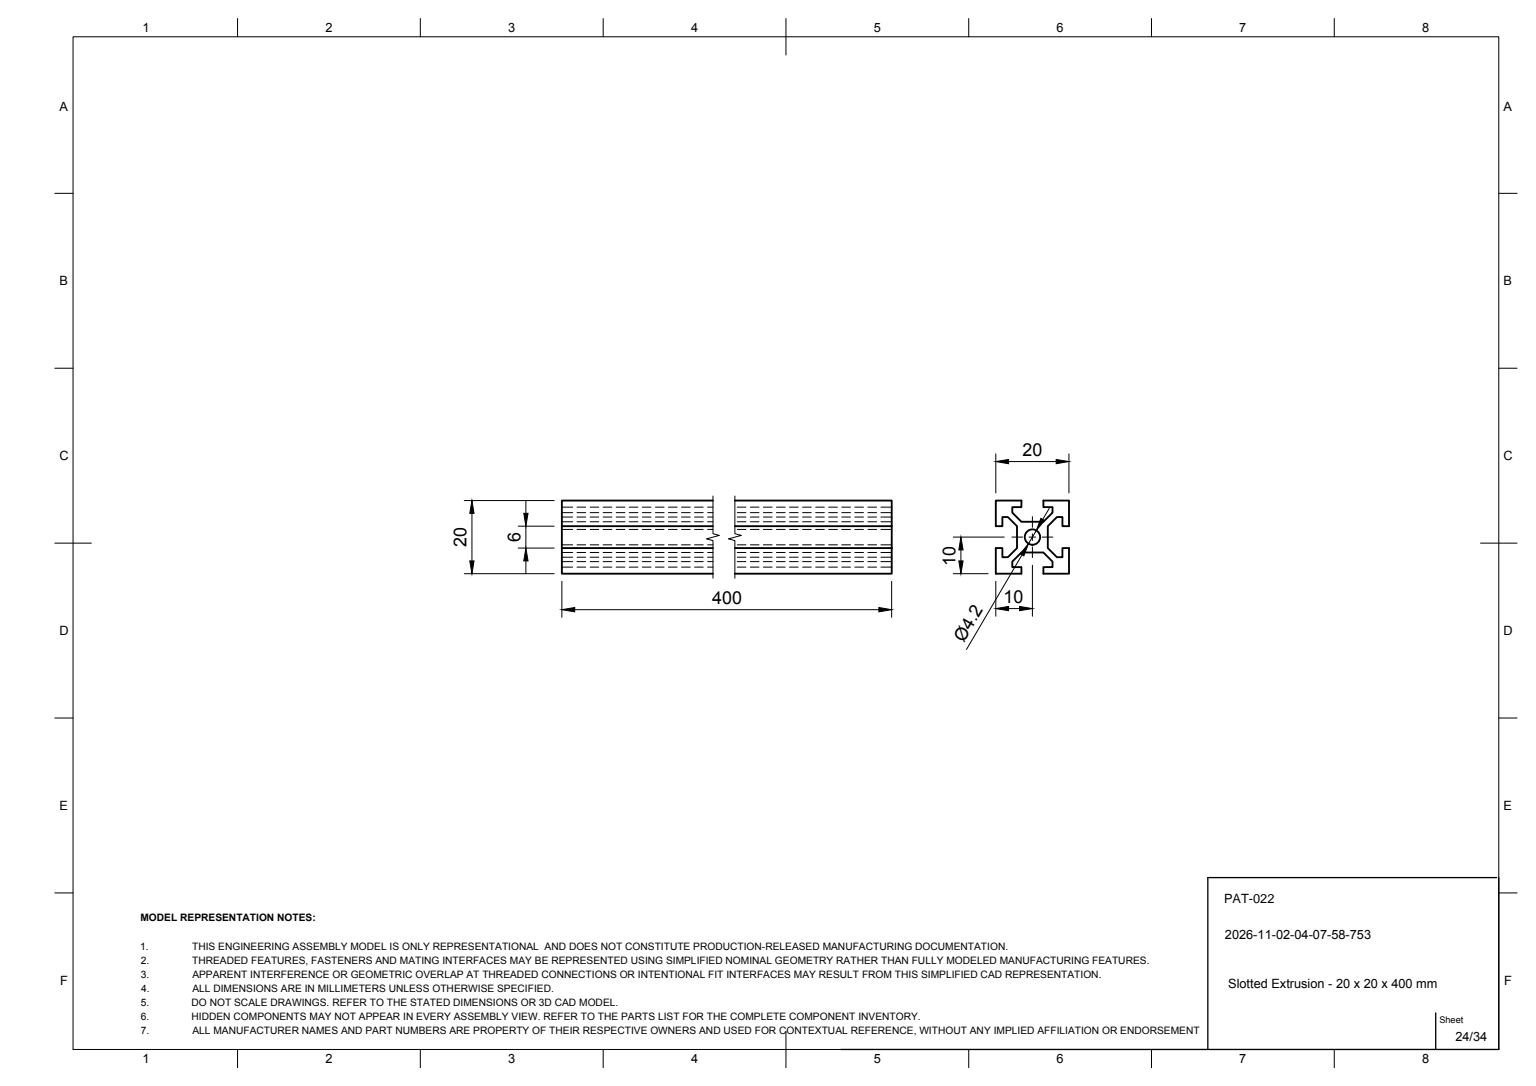
ISO-10303-21;
HEADER;
/* Generated by software containing ST-Developer
 * from STEP Tools, Inc. (www.steptools.com) 
 */

FILE_DESCRIPTION(
/* description */ ('Chute with adjustable gate'),
/* implementation_level */ '2;1');

FILE_NAME(
/* name */ 'Slotted Extrusion - 20 x 20 x 400 mm.step',
/* time_stamp */ '2026-10-27T10:52:28-07:00',
/* author */ (''),
/* organization */ (''),
/* preprocessor_version */ 'ST-DEVELOPER v20.2',
/* originating_system */ 'Autodesk Translation Framework v15.17.0.0',
/* authorisation */ '');

FILE_SCHEMA (('AUTOMOTIVE_DESIGN { 1 0 10303 214 3 1 1 }'));
ENDSEC;

DATA;
#10=MECHANICAL_DESIGN_GEOMETRIC_PRESENTATION_REPRESENTATION('',(#433),#13094);
#369=SHAPE_REPRESENTATION_RELATIONSHIP('SRR','None',#13270,#401);
#401=ADVANCED_BREP_SHAPE_REPRESENTATION('',(#465),#13079);
#433=STYLED_ITEM('',(#13481),#465);
#465=MANIFOLD_SOLID_BREP('Body1',#7616);
#550=FACE_BOUND('',#1635,.T.);
#551=FACE_BOUND('',#1637,.T.);
#734=PLANE('',#8272);
#735=PLANE('',#8273);
#736=PLANE('',#8274);
#737=PLANE('',#8275);
#738=PLANE('',#8276);
#739=PLANE('',#8277);
#740=PLANE('',#8278);
#741=PLANE('',#8279);
#742=PLANE('',#8280);
#743=PLANE('',#8281);
#744=PLANE('',#8282);
#745=PLANE('',#8283);
#746=PLANE('',#8284);
#747=PLANE('',#8285);
#748=PLANE('',#8286);
#749=PLANE('',#8287);
#750=PLANE('',#8288);
#751=PLANE('',#8289);
#752=PLANE('',#8290);
#753=PLANE('',#8291);
#754=PLANE('',#8292);
#755=PLANE('',#8293);
#756=PLANE('',#8294);
#757=PLANE('',#8295);
#758=PLANE('',#8296);
#759=PLANE('',#8297);
#760=PLANE('',#8298);
#761=PLANE('',#8299);
#762=PLANE('',#8300);
#763=PLANE('',#8301);
#764=PLANE('',#8302);
#765=PLANE('',#8303);
#766=PLANE('',#8304);
#767=PLANE('',#8305);
#768=PLANE('',#8306);
#769=PLANE('',#8307);
#770=PLANE('',#8311);
#771=PLANE('',#8312);
#772=PLANE('',#8313);
#773=PLANE('',#8314);
#774=PLANE('',#8315);
#775=PLANE('',#8316);
#776=PLANE('',#8317);
#777=PLANE('',#8318);
#778=PLANE('',#8319);
#779=PLANE('',#8320);
#1098=FACE_OUTER_BOUND('',#1589,.T.);
#1099=FACE_OUTER_BOUND('',#1590,.T.);
#1100=FACE_OUTER_BOUND('',#1591,.T.);
#1101=FACE_OUTER_BOUND('',#1592,.T.);
#1102=FACE_OUTER_BOUND('',#1593,.T.);
#1103=FACE_OUTER_BOUND('',#1594,.T.);
#1104=FACE_OUTER_BOUND('',#1595,.T.);
#1105=FACE_OUTER_BOUND('',#1596,.T.);
#1106=FACE_OUTER_BOUND('',#1597,.T.);
#1107=FACE_OUTER_BOUND('',#1598,.T.);
#1108=FACE_OUTER_BOUND('',#1599,.T.);
#1109=FACE_OUTER_BOUND('',#1600,.T.);
#1110=FACE_OUTER_BOUND('',#1601,.T.);
#1111=FACE_OUTER_BOUND('',#1602,.T.);
#1112=FACE_OUTER_BOUND('',#1603,.T.);
#1113=FACE_OUTER_BOUND('',#1604,.T.);
#1114=FACE_OUTER_BOUND('',#1605,.T.);
#1115=FACE_OUTER_BOUND('',#1606,.T.);
#1116=FACE_OUTER_BOUND('',#1607,.T.);
#1117=FACE_OUTER_BOUND('',#1608,.T.);
#1118=FACE_OUTER_BOUND('',#1609,.T.);
#1119=FACE_OUTER_BOUND('',#1610,.T.);
#1120=FACE_OUTER_BOUND('',#1611,.T.);
#1121=FACE_OUTER_BOUND('',#1612,.T.);
#1122=FACE_OUTER_BOUND('',#1613,.T.);
#1123=FACE_OUTER_BOUND('',#1614,.T.);
#1124=FACE_OUTER_BOUND('',#1615,.T.);
#1125=FACE_OUTER_BOUND('',#1616,.T.);
#1126=FACE_OUTER_BOUND('',#1617,.T.);
#1127=FACE_OUTER_BOUND('',#1618,.T.);
#1128=FACE_OUTER_BOUND('',#1619,.T.);
#1129=FACE_OUTER_BOUND('',#1620,.T.);
#1130=FACE_OUTER_BOUND('',#1621,.T.);
#1131=FACE_OUTER_BOUND('',#1622,.T.);
#1132=FACE_OUTER_BOUND('',#1623,.T.);
#1133=FACE_OUTER_BOUND('',#1624,.T.);
#1134=FACE_OUTER_BOUND('',#1625,.T.);
#1135=FACE_OUTER_BOUND('',#1626,.T.);
#1136=FACE_OUTER_BOUND('',#1627,.T.);
#1137=FACE_OUTER_BOUND('',#1628,.T.);
#1138=FACE_OUTER_BOUND('',#1629,.T.);
#1139=FACE_OUTER_BOUND('',#1630,.T.);
#1140=FACE_OUTER_BOUND('',#1631,.T.);
#1141=FACE_OUTER_BOUND('',#1632,.T.);
#1142=FACE_OUTER_BOUND('',#1633,.T.);
#1143=FACE_OUTER_BOUND('',#1634,.T.);
#1144=FACE_OUTER_BOUND('',#1636,.T.);
#1589=EDGE_LOOP('',(#6002,#6003,#6004,#6005));
#1590=EDGE_LOOP('',(#6006,#6007,#6008,#6009));
#1591=EDGE_LOOP('',(#6010,#6011,#6012,#6013));
#1592=EDGE_LOOP('',(#6014,#6015,#6016,#6017));
#1593=EDGE_LOOP('',(#6018,#6019,#6020,#6021));
#1594=EDGE_LOOP('',(#6022,#6023,#6024,#6025));
#1595=EDGE_LOOP('',(#6026,#6027,#6028,#6029));
#1596=EDGE_LOOP('',(#6030,#6031,#6032,#6033));
#1597=EDGE_LOOP('',(#6034,#6035,#6036,#6037));
#1598=EDGE_LOOP('',(#6038,#6039,#6040,#6041));
#1599=EDGE_LOOP('',(#6042,#6043,#6044,#6045));
#1600=EDGE_LOOP('',(#6046,#6047,#6048,#6049));
#1601=EDGE_LOOP('',(#6050,#6051,#6052,#6053));
#1602=EDGE_LOOP('',(#6054,#6055,#6056,#6057));
#1603=EDGE_LOOP('',(#6058,#6059,#6060,#6061));
#1604=EDGE_LOOP('',(#6062,#6063,#6064,#6065));
#1605=EDGE_LOOP('',(#6066,#6067,#6068,#6069));
#1606=EDGE_LOOP('',(#6070,#6071,#6072,#6073));
#1607=EDGE_LOOP('',(#6074,#6075,#6076,#6077));
#1608=EDGE_LOOP('',(#6078,#6079,#6080,#6081));
#1609=EDGE_LOOP('',(#6082,#6083,#6084,#6085));
#1610=EDGE_LOOP('',(#6086,#6087,#6088,#6089));
#1611=EDGE_LOOP('',(#6090,#6091,#6092,#6093));
#1612=EDGE_LOOP('',(#6094,#6095,#6096,#6097));
#1613=EDGE_LOOP('',(#6098,#6099,#6100,#6101));
#1614=EDGE_LOOP('',(#6102,#6103,#6104,#6105));
#1615=EDGE_LOOP('',(#6106,#6107,#6108,#6109));
#1616=EDGE_LOOP('',(#6110,#6111,#6112,#6113));
#1617=EDGE_LOOP('',(#6114,#6115,#6116,#6117));
#1618=EDGE_LOOP('',(#6118,#6119,#6120,#6121));
#1619=EDGE_LOOP('',(#6122,#6123,#6124,#6125));
#1620=EDGE_LOOP('',(#6126,#6127,#6128,#6129));
#1621=EDGE_LOOP('',(#6130,#6131,#6132,#6133));
#1622=EDGE_LOOP('',(#6134,#6135,#6136,#6137));
#1623=EDGE_LOOP('',(#6138,#6139,#6140,#6141));
#1624=EDGE_LOOP('',(#6142,#6143,#6144,#6145));
#1625=EDGE_LOOP('',(#6146,#6147,#6148,#6149));
#1626=EDGE_LOOP('',(#6150,#6151,#6152,#6153));
#1627=EDGE_LOOP('',(#6154,#6155,#6156,#6157));
#1628=EDGE_LOOP('',(#6158,#6159,#6160,#6161));
#1629=EDGE_LOOP('',(#6162,#6163,#6164,#6165));
#1630=EDGE_LOOP('',(#6166,#6167,#6168,#6169));
#1631=EDGE_LOOP('',(#6170,#6171,#6172,#6173));
#1632=EDGE_LOOP('',(#6174,#6175,#6176,#6177));
#1633=EDGE_LOOP('',(#6178,#6179,#6180,#6181));
#1634=EDGE_LOOP('',(#6182,#6183,#6184,#6185,#6186,#6187,#6188,#6189,#6190,
#6191,#6192,#6193,#6194,#6195,#6196,#6197,#6198,#6199,#6200,#6201,#6202,
#6203,#6204,#6205,#6206,#6207,#6208,#6209,#6210,#6211,#6212,#6213,#6214,
#6215,#6216,#6217,#6218,#6219,#6220,#6221,#6222,#6223,#6224,#6225));
#1635=EDGE_LOOP('',(#6226));
#1636=EDGE_LOOP('',(#6227,#6228,#6229,#6230,#6231,#6232,#6233,#6234,#6235,
#6236,#6237,#6238,#6239,#6240,#6241,#6242,#6243,#6244,#6245,#6246,#6247,
#6248,#6249,#6250,#6251,#6252,#6253,#6254,#6255,#6256,#6257,#6258,#6259,
#6260,#6261,#6262,#6263,#6264,#6265,#6266,#6267,#6268,#6269,#6270));
#1637=EDGE_LOOP('',(#6271));
#2188=LINE('',#11788,#2965);
#2189=LINE('',#11790,#2966);
#2190=LINE('',#11792,#2967);
#2191=LINE('',#11793,#2968);
#2192=LINE('',#11796,#2969);
#2193=LINE('',#11798,#2970);
#2194=LINE('',#11799,#2971);
#2195=LINE('',#11802,#2972);
#2196=LINE('',#11804,#2973);
#2197=LINE('',#11805,#2974);
#2198=LINE('',#11808,#2975);
#2199=LINE('',#11810,#2976);
#2200=LINE('',#11811,#2977);
#2201=LINE('',#11814,#2978);
#2202=LINE('',#11816,#2979);
#2203=LINE('',#11817,#2980);
#2204=LINE('',#11820,#2981);
#2205=LINE('',#11822,#2982);
#2206=LINE('',#11823,#2983);
#2207=LINE('',#11826,#2984);
#2208=LINE('',#11828,#2985);
#2209=LINE('',#11829,#2986);
#2210=LINE('',#11832,#2987);
#2211=LINE('',#11834,#2988);
#2212=LINE('',#11835,#2989);
#2213=LINE('',#11838,#2990);
#2214=LINE('',#11840,#2991);
#2215=LINE('',#11841,#2992);
#2216=LINE('',#11845,#2993);
#2217=LINE('',#11847,#2994);
#2218=LINE('',#11849,#2995);
#2219=LINE('',#11850,#2996);
#2220=LINE('',#11853,#2997);
#2221=LINE('',#11855,#2998);
#2222=LINE('',#11856,#2999);
#2223=LINE('',#11859,#3000);
#2224=LINE('',#11861,#3001);
#2225=LINE('',#11862,#3002);
#2226=LINE('',#11865,#3003);
#2227=LINE('',#11867,#3004);
#2228=LINE('',#11868,#3005);
#2229=LINE('',#11871,#3006);
#2230=LINE('',#11873,#3007);
#2231=LINE('',#11874,#3008);
#2232=LINE('',#11877,#3009);
#2233=LINE('',#11879,#3010);
#2234=LINE('',#11880,#3011);
#2235=LINE('',#11883,#3012);
#2236=LINE('',#11885,#3013);
#2237=LINE('',#11886,#3014);
#2238=LINE('',#11889,#3015);
#2239=LINE('',#11891,#3016);
#2240=LINE('',#11892,#3017);
#2241=LINE('',#11895,#3018);
#2242=LINE('',#11897,#3019);
#2243=LINE('',#11898,#3020);
#2244=LINE('',#11902,#3021);
#2245=LINE('',#11904,#3022);
#2246=LINE('',#11906,#3023);
#2247=LINE('',#11907,#3024);
#2248=LINE('',#11910,#3025);
#2249=LINE('',#11912,#3026);
#2250=LINE('',#11913,#3027);
#2251=LINE('',#11916,#3028);
#2252=LINE('',#11918,#3029);
#2253=LINE('',#11919,#3030);
#2254=LINE('',#11922,#3031);
#2255=LINE('',#11924,#3032);
#2256=LINE('',#11925,#3033);
#2257=LINE('',#11928,#3034);
#2258=LINE('',#11930,#3035);
#2259=LINE('',#11931,#3036);
#2260=LINE('',#11934,#3037);
#2261=LINE('',#11936,#3038);
#2262=LINE('',#11937,#3039);
#2263=LINE('',#11940,#3040);
#2264=LINE('',#11942,#3041);
#2265=LINE('',#11943,#3042);
#2266=LINE('',#11946,#3043);
#2267=LINE('',#11948,#3044);
#2268=LINE('',#11949,#3045);
#2269=LINE('',#11952,#3046);
#2270=LINE('',#11954,#3047);
#2271=LINE('',#11955,#3048);
#2272=LINE('',#11959,#3049);
#2273=LINE('',#11961,#3050);
#2274=LINE('',#11963,#3051);
#2275=LINE('',#11964,#3052);
#2276=LINE('',#11967,#3053);
#2277=LINE('',#11969,#3054);
#2278=LINE('',#11970,#3055);
#2279=LINE('',#11973,#3056);
#2280=LINE('',#11975,#3057);
#2281=LINE('',#11976,#3058);
#2282=LINE('',#11979,#3059);
#2283=LINE('',#11981,#3060);
#2284=LINE('',#11982,#3061);
#2285=LINE('',#11985,#3062);
#2286=LINE('',#11987,#3063);
#2287=LINE('',#11988,#3064);
#2288=LINE('',#11991,#3065);
#2289=LINE('',#11993,#3066);
#2290=LINE('',#11994,#3067);
#2291=LINE('',#11997,#3068);
#2292=LINE('',#11999,#3069);
#2293=LINE('',#12000,#3070);
#2294=LINE('',#12003,#3071);
#2295=LINE('',#12005,#3072);
#2296=LINE('',#12006,#3073);
#2297=LINE('',#12009,#3074);
#2298=LINE('',#12011,#3075);
#2299=LINE('',#12012,#3076);
#2300=LINE('',#12017,#3077);
#2301=LINE('',#12021,#3078);
#2302=LINE('',#12023,#3079);
#2303=LINE('',#12024,#3080);
#2304=LINE('',#12027,#3081);
#2305=LINE('',#12029,#3082);
#2306=LINE('',#12030,#3083);
#2307=LINE('',#12032,#3084);
#2308=LINE('',#12033,#3085);
#2309=LINE('',#12036,#3086);
#2310=LINE('',#12038,#3087);
#2311=LINE('',#12039,#3088);
#2312=LINE('',#12041,#3089);
#2313=LINE('',#12042,#3090);
#2314=LINE('',#12045,#3091);
#2315=LINE('',#12047,#3092);
#2316=LINE('',#12048,#3093);
#2317=LINE('',#12050,#3094);
#2318=LINE('',#12051,#3095);
#2319=LINE('',#12053,#3096);
#2320=LINE('',#12054,#3097);
#2965=VECTOR('',#9600,1.);
#2966=VECTOR('',#9601,1.);
#2967=VECTOR('',#9602,1.);
#2968=VECTOR('',#9603,1.);
#2969=VECTOR('',#9606,1.);
#2970=VECTOR('',#9607,1.);
#2971=VECTOR('',#9608,1.);
#2972=VECTOR('',#9611,1.);
#2973=VECTOR('',#9612,1.);
#2974=VECTOR('',#9613,1.);
#2975=VECTOR('',#9616,1.);
#2976=VECTOR('',#9617,1.);
#2977=VECTOR('',#9618,1.);
#2978=VECTOR('',#9621,1.);
#2979=VECTOR('',#9622,1.);
#2980=VECTOR('',#9623,1.);
#2981=VECTOR('',#9626,1.);
#2982=VECTOR('',#9627,1.);
#2983=VECTOR('',#9628,1.);
#2984=VECTOR('',#9631,1.);
#2985=VECTOR('',#9632,1.);
#2986=VECTOR('',#9633,1.);
#2987=VECTOR('',#9636,1.);
#2988=VECTOR('',#9637,1.);
#2989=VECTOR('',#9638,1.);
#2990=VECTOR('',#9641,1.);
#2991=VECTOR('',#9642,1.);
#2992=VECTOR('',#9643,1.);
#2993=VECTOR('',#9646,1.);
#2994=VECTOR('',#9647,1.);
#2995=VECTOR('',#9648,1.);
#2996=VECTOR('',#9649,1.);
#2997=VECTOR('',#9652,1.);
#2998=VECTOR('',#9653,1.);
#2999=VECTOR('',#9654,1.);
#3000=VECTOR('',#9657,1.);
#3001=VECTOR('',#9658,1.);
#3002=VECTOR('',#9659,1.);
#3003=VECTOR('',#9662,1.);
#3004=VECTOR('',#9663,1.);
#3005=VECTOR('',#9664,1.);
#3006=VECTOR('',#9667,1.);
#3007=VECTOR('',#9668,1.);
#3008=VECTOR('',#9669,1.);
#3009=VECTOR('',#9672,1.);
#3010=VECTOR('',#9673,1.);
#3011=VECTOR('',#9674,1.);
#3012=VECTOR('',#9677,1.);
#3013=VECTOR('',#9678,1.);
#3014=VECTOR('',#9679,1.);
#3015=VECTOR('',#9682,1.);
#3016=VECTOR('',#9683,1.);
#3017=VECTOR('',#9684,1.);
#3018=VECTOR('',#9687,1.);
#3019=VECTOR('',#9688,1.);
#3020=VECTOR('',#9689,1.);
#3021=VECTOR('',#9692,1.);
#3022=VECTOR('',#9693,1.);
#3023=VECTOR('',#9694,1.);
#3024=VECTOR('',#9695,1.);
#3025=VECTOR('',#9698,1.);
#3026=VECTOR('',#9699,1.);
#3027=VECTOR('',#9700,1.);
#3028=VECTOR('',#9703,1.);
#3029=VECTOR('',#9704,1.);
#3030=VECTOR('',#9705,1.);
#3031=VECTOR('',#9708,1.);
#3032=VECTOR('',#9709,1.);
#3033=VECTOR('',#9710,1.);
#3034=VECTOR('',#9713,1.);
#3035=VECTOR('',#9714,1.);
#3036=VECTOR('',#9715,1.);
#3037=VECTOR('',#9718,1.);
#3038=VECTOR('',#9719,1.);
#3039=VECTOR('',#9720,1.);
#3040=VECTOR('',#9723,1.);
#3041=VECTOR('',#9724,1.);
#3042=VECTOR('',#9725,1.);
#3043=VECTOR('',#9728,1.);
#3044=VECTOR('',#9729,1.);
#3045=VECTOR('',#9730,1.);
#3046=VECTOR('',#9733,1.);
#3047=VECTOR('',#9734,1.);
#3048=VECTOR('',#9735,1.);
#3049=VECTOR('',#9738,1.);
#3050=VECTOR('',#9739,1.);
#3051=VECTOR('',#9740,1.);
#3052=VECTOR('',#9741,1.);
#3053=VECTOR('',#9744,1.);
#3054=VECTOR('',#9745,1.);
#3055=VECTOR('',#9746,1.);
#3056=VECTOR('',#9749,1.);
#3057=VECTOR('',#9750,1.);
#3058=VECTOR('',#9751,1.);
#3059=VECTOR('',#9754,1.);
#3060=VECTOR('',#9755,1.);
#3061=VECTOR('',#9756,1.);
#3062=VECTOR('',#9759,1.);
#3063=VECTOR('',#9760,1.);
#3064=VECTOR('',#9761,1.);
#3065=VECTOR('',#9764,1.);
#3066=VECTOR('',#9765,1.);
#3067=VECTOR('',#9766,1.);
#3068=VECTOR('',#9769,1.);
#3069=VECTOR('',#9770,1.);
#3070=VECTOR('',#9771,1.);
#3071=VECTOR('',#9774,1.);
#3072=VECTOR('',#9775,1.);
#3073=VECTOR('',#9776,1.);
#3074=VECTOR('',#9779,1.);
#3075=VECTOR('',#9780,1.);
#3076=VECTOR('',#9781,1.);
#3077=VECTOR('',#9786,0.21);
#3078=VECTOR('',#9791,1.);
#3079=VECTOR('',#9792,1.);
#3080=VECTOR('',#9793,1.);
#3081=VECTOR('',#9796,1.);
#3082=VECTOR('',#9797,1.);
#3083=VECTOR('',#9798,1.);
#3084=VECTOR('',#9801,1.);
#3085=VECTOR('',#9802,1.);
#3086=VECTOR('',#9805,1.);
#3087=VECTOR('',#9806,1.);
#3088=VECTOR('',#9807,1.);
#3089=VECTOR('',#9810,1.);
#3090=VECTOR('',#9811,1.);
#3091=VECTOR('',#9814,1.);
#3092=VECTOR('',#9815,1.);
#3093=VECTOR('',#9816,1.);
#3094=VECTOR('',#9819,1.);
#3095=VECTOR('',#9820,1.);
#3096=VECTOR('',#9823,1.);
#3097=VECTOR('',#9824,1.);
#3494=CIRCLE('',#8309,0.21);
#3495=CIRCLE('',#8310,0.21);
#3865=VERTEX_POINT('',#11786);
#3866=VERTEX_POINT('',#11787);
#3867=VERTEX_POINT('',#11789);
#3868=VERTEX_POINT('',#11791);
#3869=VERTEX_POINT('',#11795);
#3870=VERTEX_POINT('',#11797);
#3871=VERTEX_POINT('',#11801);
#3872=VERTEX_POINT('',#11803);
#3873=VERTEX_POINT('',#11807);
#3874=VERTEX_POINT('',#11809);
#3875=VERTEX_POINT('',#11813);
#3876=VERTEX_POINT('',#11815);
#3877=VERTEX_POINT('',#11819);
#3878=VERTEX_POINT('',#11821);
#3879=VERTEX_POINT('',#11825);
#3880=VERTEX_POINT('',#11827);
#3881=VERTEX_POINT('',#11831);
#3882=VERTEX_POINT('',#11833);
#3883=VERTEX_POINT('',#11837);
#3884=VERTEX_POINT('',#11839);
#3885=VERTEX_POINT('',#11843);
#3886=VERTEX_POINT('',#11844);
#3887=VERTEX_POINT('',#11846);
#3888=VERTEX_POINT('',#11848);
#3889=VERTEX_POINT('',#11852);
#3890=VERTEX_POINT('',#11854);
#3891=VERTEX_POINT('',#11858);
#3892=VERTEX_POINT('',#11860);
#3893=VERTEX_POINT('',#11864);
#3894=VERTEX_POINT('',#11866);
#3895=VERTEX_POINT('',#11870);
#3896=VERTEX_POINT('',#11872);
#3897=VERTEX_POINT('',#11876);
#3898=VERTEX_POINT('',#11878);
#3899=VERTEX_POINT('',#11882);
#3900=VERTEX_POINT('',#11884);
#3901=VERTEX_POINT('',#11888);
#3902=VERTEX_POINT('',#11890);
#3903=VERTEX_POINT('',#11894);
#3904=VERTEX_POINT('',#11896);
#3905=VERTEX_POINT('',#11900);
#3906=VERTEX_POINT('',#11901);
#3907=VERTEX_POINT('',#11903);
#3908=VERTEX_POINT('',#11905);
#3909=VERTEX_POINT('',#11909);
#3910=VERTEX_POINT('',#11911);
#3911=VERTEX_POINT('',#11915);
#3912=VERTEX_POINT('',#11917);
#3913=VERTEX_POINT('',#11921);
#3914=VERTEX_POINT('',#11923);
#3915=VERTEX_POINT('',#11927);
#3916=VERTEX_POINT('',#11929);
#3917=VERTEX_POINT('',#11933);
#3918=VERTEX_POINT('',#11935);
#3919=VERTEX_POINT('',#11939);
#3920=VERTEX_POINT('',#11941);
#3921=VERTEX_POINT('',#11945);
#3922=VERTEX_POINT('',#11947);
#3923=VERTEX_POINT('',#11951);
#3924=VERTEX_POINT('',#11953);
#3925=VERTEX_POINT('',#11957);
#3926=VERTEX_POINT('',#11958);
#3927=VERTEX_POINT('',#11960);
#3928=VERTEX_POINT('',#11962);
#3929=VERTEX_POINT('',#11966);
#3930=VERTEX_POINT('',#11968);
#3931=VERTEX_POINT('',#11972);
#3932=VERTEX_POINT('',#11974);
#3933=VERTEX_POINT('',#11978);
#3934=VERTEX_POINT('',#11980);
#3935=VERTEX_POINT('',#11984);
#3936=VERTEX_POINT('',#11986);
#3937=VERTEX_POINT('',#11990);
#3938=VERTEX_POINT('',#11992);
#3939=VERTEX_POINT('',#11996);
#3940=VERTEX_POINT('',#11998);
#3941=VERTEX_POINT('',#12002);
#3942=VERTEX_POINT('',#12004);
#3943=VERTEX_POINT('',#12008);
#3944=VERTEX_POINT('',#12010);
#3945=VERTEX_POINT('',#12014);
#3946=VERTEX_POINT('',#12016);
#3947=VERTEX_POINT('',#12020);
#3948=VERTEX_POINT('',#12022);
#3949=VERTEX_POINT('',#12026);
#3950=VERTEX_POINT('',#12028);
#3951=VERTEX_POINT('',#12035);
#3952=VERTEX_POINT('',#12037);
#3953=VERTEX_POINT('',#12044);
#3954=VERTEX_POINT('',#12046);
#4634=EDGE_CURVE('',#3865,#3866,#2188,.T.);
#4635=EDGE_CURVE('',#3865,#3867,#2189,.T.);
#4636=EDGE_CURVE('',#3868,#3867,#2190,.T.);
#4637=EDGE_CURVE('',#3866,#3868,#2191,.T.);
#4638=EDGE_CURVE('',#3869,#3865,#2192,.T.);
#4639=EDGE_CURVE('',#3869,#3870,#2193,.T.);
#4640=EDGE_CURVE('',#3867,#3870,#2194,.T.);
#4641=EDGE_CURVE('',#3871,#3869,#2195,.T.);
#4642=EDGE_CURVE('',#3871,#3872,#2196,.T.);
#4643=EDGE_CURVE('',#3870,#3872,#2197,.T.);
#4644=EDGE_CURVE('',#3873,#3871,#2198,.T.);
#4645=EDGE_CURVE('',#3873,#3874,#2199,.T.);
#4646=EDGE_CURVE('',#3872,#3874,#2200,.T.);
#4647=EDGE_CURVE('',#3875,#3873,#2201,.T.);
#4648=EDGE_CURVE('',#3875,#3876,#2202,.T.);
#4649=EDGE_CURVE('',#3874,#3876,#2203,.T.);
#4650=EDGE_CURVE('',#3877,#3875,#2204,.T.);
#4651=EDGE_CURVE('',#3877,#3878,#2205,.T.);
#4652=EDGE_CURVE('',#3876,#3878,#2206,.T.);
#4653=EDGE_CURVE('',#3879,#3877,#2207,.T.);
#4654=EDGE_CURVE('',#3879,#3880,#2208,.T.);
#4655=EDGE_CURVE('',#3878,#3880,#2209,.T.);
#4656=EDGE_CURVE('',#3881,#3879,#2210,.T.);
#4657=EDGE_CURVE('',#3881,#3882,#2211,.T.);
#4658=EDGE_CURVE('',#3880,#3882,#2212,.T.);
#4659=EDGE_CURVE('',#3883,#3881,#2213,.T.);
#4660=EDGE_CURVE('',#3884,#3883,#2214,.T.);
#4661=EDGE_CURVE('',#3882,#3884,#2215,.T.);
#4662=EDGE_CURVE('',#3885,#3886,#2216,.T.);
#4663=EDGE_CURVE('',#3885,#3887,#2217,.T.);
#4664=EDGE_CURVE('',#3888,#3887,#2218,.T.);
#4665=EDGE_CURVE('',#3886,#3888,#2219,.T.);
#4666=EDGE_CURVE('',#3889,#3885,#2220,.T.);
#4667=EDGE_CURVE('',#3889,#3890,#2221,.T.);
#4668=EDGE_CURVE('',#3887,#3890,#2222,.T.);
#4669=EDGE_CURVE('',#3891,#3889,#2223,.T.);
#4670=EDGE_CURVE('',#3891,#3892,#2224,.T.);
#4671=EDGE_CURVE('',#3890,#3892,#2225,.T.);
#4672=EDGE_CURVE('',#3893,#3891,#2226,.T.);
#4673=EDGE_CURVE('',#3893,#3894,#2227,.T.);
#4674=EDGE_CURVE('',#3892,#3894,#2228,.T.);
#4675=EDGE_CURVE('',#3895,#3893,#2229,.T.);
#4676=EDGE_CURVE('',#3895,#3896,#2230,.T.);
#4677=EDGE_CURVE('',#3894,#3896,#2231,.T.);
#4678=EDGE_CURVE('',#3897,#3895,#2232,.T.);
#4679=EDGE_CURVE('',#3897,#3898,#2233,.T.);
#4680=EDGE_CURVE('',#3896,#3898,#2234,.T.);
#4681=EDGE_CURVE('',#3899,#3897,#2235,.T.);
#4682=EDGE_CURVE('',#3899,#3900,#2236,.T.);
#4683=EDGE_CURVE('',#3898,#3900,#2237,.T.);
#4684=EDGE_CURVE('',#3901,#3899,#2238,.T.);
#4685=EDGE_CURVE('',#3901,#3902,#2239,.T.);
#4686=EDGE_CURVE('',#3900,#3902,#2240,.T.);
#4687=EDGE_CURVE('',#3903,#3901,#2241,.T.);
#4688=EDGE_CURVE('',#3904,#3903,#2242,.T.);
#4689=EDGE_CURVE('',#3902,#3904,#2243,.T.);
#4690=EDGE_CURVE('',#3905,#3906,#2244,.T.);
#4691=EDGE_CURVE('',#3905,#3907,#2245,.T.);
#4692=EDGE_CURVE('',#3908,#3907,#2246,.T.);
#4693=EDGE_CURVE('',#3906,#3908,#2247,.T.);
#4694=EDGE_CURVE('',#3909,#3905,#2248,.T.);
#4695=EDGE_CURVE('',#3909,#3910,#2249,.T.);
#4696=EDGE_CURVE('',#3907,#3910,#2250,.T.);
#4697=EDGE_CURVE('',#3911,#3909,#2251,.T.);
#4698=EDGE_CURVE('',#3911,#3912,#2252,.T.);
#4699=EDGE_CURVE('',#3910,#3912,#2253,.T.);
#4700=EDGE_CURVE('',#3913,#3911,#2254,.T.);
#4701=EDGE_CURVE('',#3913,#3914,#2255,.T.);
#4702=EDGE_CURVE('',#3912,#3914,#2256,.T.);
#4703=EDGE_CURVE('',#3915,#3913,#2257,.T.);
#4704=EDGE_CURVE('',#3915,#3916,#2258,.T.);
#4705=EDGE_CURVE('',#3914,#3916,#2259,.T.);
#4706=EDGE_CURVE('',#3917,#3915,#2260,.T.);
#4707=EDGE_CURVE('',#3917,#3918,#2261,.T.);
#4708=EDGE_CURVE('',#3916,#3918,#2262,.T.);
#4709=EDGE_CURVE('',#3919,#3917,#2263,.T.);
#4710=EDGE_CURVE('',#3919,#3920,#2264,.T.);
#4711=EDGE_CURVE('',#3918,#3920,#2265,.T.);
#4712=EDGE_CURVE('',#3921,#3919,#2266,.T.);
#4713=EDGE_CURVE('',#3921,#3922,#2267,.T.);
#4714=EDGE_CURVE('',#3920,#3922,#2268,.T.);
#4715=EDGE_CURVE('',#3923,#3921,#2269,.T.);
#4716=EDGE_CURVE('',#3924,#3923,#2270,.T.);
#4717=EDGE_CURVE('',#3922,#3924,#2271,.T.);
#4718=EDGE_CURVE('',#3925,#3926,#2272,.T.);
#4719=EDGE_CURVE('',#3925,#3927,#2273,.T.);
#4720=EDGE_CURVE('',#3928,#3927,#2274,.T.);
#4721=EDGE_CURVE('',#3926,#3928,#2275,.T.);
#4722=EDGE_CURVE('',#3929,#3925,#2276,.T.);
#4723=EDGE_CURVE('',#3929,#3930,#2277,.T.);
#4724=EDGE_CURVE('',#3927,#3930,#2278,.T.);
#4725=EDGE_CURVE('',#3931,#3929,#2279,.T.);
#4726=EDGE_CURVE('',#3931,#3932,#2280,.T.);
#4727=EDGE_CURVE('',#3930,#3932,#2281,.T.);
#4728=EDGE_CURVE('',#3933,#3931,#2282,.T.);
#4729=EDGE_CURVE('',#3933,#3934,#2283,.T.);
#4730=EDGE_CURVE('',#3932,#3934,#2284,.T.);
#4731=EDGE_CURVE('',#3935,#3933,#2285,.T.);
#4732=EDGE_CURVE('',#3935,#3936,#2286,.T.);
#4733=EDGE_CURVE('',#3934,#3936,#2287,.T.);
#4734=EDGE_CURVE('',#3937,#3935,#2288,.T.);
#4735=EDGE_CURVE('',#3937,#3938,#2289,.T.);
#4736=EDGE_CURVE('',#3936,#3938,#2290,.T.);
#4737=EDGE_CURVE('',#3939,#3937,#2291,.T.);
#4738=EDGE_CURVE('',#3939,#3940,#2292,.T.);
#4739=EDGE_CURVE('',#3938,#3940,#2293,.T.);
#4740=EDGE_CURVE('',#3941,#3939,#2294,.T.);
#4741=EDGE_CURVE('',#3941,#3942,#2295,.T.);
#4742=EDGE_CURVE('',#3940,#3942,#2296,.T.);
#4743=EDGE_CURVE('',#3943,#3941,#2297,.T.);
#4744=EDGE_CURVE('',#3944,#3943,#2298,.T.);
#4745=EDGE_CURVE('',#3942,#3944,#2299,.T.);
#4746=EDGE_CURVE('',#3945,#3945,#3494,.T.);
#4747=EDGE_CURVE('',#3945,#3946,#2300,.T.);
#4748=EDGE_CURVE('',#3946,#3946,#3495,.T.);
#4749=EDGE_CURVE('',#3883,#3947,#2301,.T.);
#4750=EDGE_CURVE('',#3947,#3948,#2302,.T.);
#4751=EDGE_CURVE('',#3884,#3948,#2303,.T.);
#4752=EDGE_CURVE('',#3949,#3868,#2304,.T.);
#4753=EDGE_CURVE('',#3950,#3949,#2305,.T.);
#4754=EDGE_CURVE('',#3950,#3866,#2306,.T.);
#4755=EDGE_CURVE('',#3903,#3950,#2307,.T.);
#4756=EDGE_CURVE('',#3904,#3949,#2308,.T.);
#4757=EDGE_CURVE('',#3951,#3888,#2309,.T.);
#4758=EDGE_CURVE('',#3952,#3951,#2310,.T.);
#4759=EDGE_CURVE('',#3952,#3886,#2311,.T.);
#4760=EDGE_CURVE('',#3923,#3952,#2312,.T.);
#4761=EDGE_CURVE('',#3924,#3951,#2313,.T.);
#4762=EDGE_CURVE('',#3953,#3908,#2314,.T.);
#4763=EDGE_CURVE('',#3954,#3953,#2315,.T.);
#4764=EDGE_CURVE('',#3954,#3906,#2316,.T.);
#4765=EDGE_CURVE('',#3943,#3954,#2317,.T.);
#4766=EDGE_CURVE('',#3944,#3953,#2318,.T.);
#4767=EDGE_CURVE('',#3948,#3928,#2319,.T.);
#4768=EDGE_CURVE('',#3947,#3926,#2320,.T.);
#6002=ORIENTED_EDGE('',*,*,#4634,.F.);
#6003=ORIENTED_EDGE('',*,*,#4635,.T.);
#6004=ORIENTED_EDGE('',*,*,#4636,.F.);
#6005=ORIENTED_EDGE('',*,*,#4637,.F.);
#6006=ORIENTED_EDGE('',*,*,#4638,.F.);
#6007=ORIENTED_EDGE('',*,*,#4639,.T.);
#6008=ORIENTED_EDGE('',*,*,#4640,.F.);
#6009=ORIENTED_EDGE('',*,*,#4635,.F.);
#6010=ORIENTED_EDGE('',*,*,#4641,.F.);
#6011=ORIENTED_EDGE('',*,*,#4642,.T.);
#6012=ORIENTED_EDGE('',*,*,#4643,.F.);
#6013=ORIENTED_EDGE('',*,*,#4639,.F.);
#6014=ORIENTED_EDGE('',*,*,#4644,.F.);
#6015=ORIENTED_EDGE('',*,*,#4645,.T.);
#6016=ORIENTED_EDGE('',*,*,#4646,.F.);
#6017=ORIENTED_EDGE('',*,*,#4642,.F.);
#6018=ORIENTED_EDGE('',*,*,#4647,.F.);
#6019=ORIENTED_EDGE('',*,*,#4648,.T.);
#6020=ORIENTED_EDGE('',*,*,#4649,.F.);
#6021=ORIENTED_EDGE('',*,*,#4645,.F.);
#6022=ORIENTED_EDGE('',*,*,#4650,.F.);
#6023=ORIENTED_EDGE('',*,*,#4651,.T.);
#6024=ORIENTED_EDGE('',*,*,#4652,.F.);
#6025=ORIENTED_EDGE('',*,*,#4648,.F.);
#6026=ORIENTED_EDGE('',*,*,#4653,.F.);
#6027=ORIENTED_EDGE('',*,*,#4654,.T.);
#6028=ORIENTED_EDGE('',*,*,#4655,.F.);
#6029=ORIENTED_EDGE('',*,*,#4651,.F.);
#6030=ORIENTED_EDGE('',*,*,#4656,.F.);
#6031=ORIENTED_EDGE('',*,*,#4657,.T.);
#6032=ORIENTED_EDGE('',*,*,#4658,.F.);
#6033=ORIENTED_EDGE('',*,*,#4654,.F.);
#6034=ORIENTED_EDGE('',*,*,#4659,.F.);
#6035=ORIENTED_EDGE('',*,*,#4660,.F.);
#6036=ORIENTED_EDGE('',*,*,#4661,.F.);
#6037=ORIENTED_EDGE('',*,*,#4657,.F.);
#6038=ORIENTED_EDGE('',*,*,#4662,.F.);
#6039=ORIENTED_EDGE('',*,*,#4663,.T.);
#6040=ORIENTED_EDGE('',*,*,#4664,.F.);
#6041=ORIENTED_EDGE('',*,*,#4665,.F.);
#6042=ORIENTED_EDGE('',*,*,#4666,.F.);
#6043=ORIENTED_EDGE('',*,*,#4667,.T.);
#6044=ORIENTED_EDGE('',*,*,#4668,.F.);
#6045=ORIENTED_EDGE('',*,*,#4663,.F.);
#6046=ORIENTED_EDGE('',*,*,#4669,.F.);
#6047=ORIENTED_EDGE('',*,*,#4670,.T.);
#6048=ORIENTED_EDGE('',*,*,#4671,.F.);
#6049=ORIENTED_EDGE('',*,*,#4667,.F.);
#6050=ORIENTED_EDGE('',*,*,#4672,.F.);
#6051=ORIENTED_EDGE('',*,*,#4673,.T.);
#6052=ORIENTED_EDGE('',*,*,#4674,.F.);
#6053=ORIENTED_EDGE('',*,*,#4670,.F.);
#6054=ORIENTED_EDGE('',*,*,#4675,.F.);
#6055=ORIENTED_EDGE('',*,*,#4676,.T.);
#6056=ORIENTED_EDGE('',*,*,#4677,.F.);
#6057=ORIENTED_EDGE('',*,*,#4673,.F.);
#6058=ORIENTED_EDGE('',*,*,#4678,.F.);
#6059=ORIENTED_EDGE('',*,*,#4679,.T.);
#6060=ORIENTED_EDGE('',*,*,#4680,.F.);
#6061=ORIENTED_EDGE('',*,*,#4676,.F.);
#6062=ORIENTED_EDGE('',*,*,#4681,.F.);
#6063=ORIENTED_EDGE('',*,*,#4682,.T.);
#6064=ORIENTED_EDGE('',*,*,#4683,.F.);
#6065=ORIENTED_EDGE('',*,*,#4679,.F.);
#6066=ORIENTED_EDGE('',*,*,#4684,.F.);
#6067=ORIENTED_EDGE('',*,*,#4685,.T.);
#6068=ORIENTED_EDGE('',*,*,#4686,.F.);
#6069=ORIENTED_EDGE('',*,*,#4682,.F.);
#6070=ORIENTED_EDGE('',*,*,#4687,.F.);
#6071=ORIENTED_EDGE('',*,*,#4688,.F.);
#6072=ORIENTED_EDGE('',*,*,#4689,.F.);
#6073=ORIENTED_EDGE('',*,*,#4685,.F.);
#6074=ORIENTED_EDGE('',*,*,#4690,.F.);
#6075=ORIENTED_EDGE('',*,*,#4691,.T.);
#6076=ORIENTED_EDGE('',*,*,#4692,.F.);
#6077=ORIENTED_EDGE('',*,*,#4693,.F.);
#6078=ORIENTED_EDGE('',*,*,#4694,.F.);
#6079=ORIENTED_EDGE('',*,*,#4695,.T.);
#6080=ORIENTED_EDGE('',*,*,#4696,.F.);
#6081=ORIENTED_EDGE('',*,*,#4691,.F.);
#6082=ORIENTED_EDGE('',*,*,#4697,.F.);
#6083=ORIENTED_EDGE('',*,*,#4698,.T.);
#6084=ORIENTED_EDGE('',*,*,#4699,.F.);
#6085=ORIENTED_EDGE('',*,*,#4695,.F.);
#6086=ORIENTED_EDGE('',*,*,#4700,.F.);
#6087=ORIENTED_EDGE('',*,*,#4701,.T.);
#6088=ORIENTED_EDGE('',*,*,#4702,.F.);
#6089=ORIENTED_EDGE('',*,*,#4698,.F.);
#6090=ORIENTED_EDGE('',*,*,#4703,.F.);
#6091=ORIENTED_EDGE('',*,*,#4704,.T.);
#6092=ORIENTED_EDGE('',*,*,#4705,.F.);
#6093=ORIENTED_EDGE('',*,*,#4701,.F.);
#6094=ORIENTED_EDGE('',*,*,#4706,.F.);
#6095=ORIENTED_EDGE('',*,*,#4707,.T.);
#6096=ORIENTED_EDGE('',*,*,#4708,.F.);
#6097=ORIENTED_EDGE('',*,*,#4704,.F.);
#6098=ORIENTED_EDGE('',*,*,#4709,.F.);
#6099=ORIENTED_EDGE('',*,*,#4710,.T.);
#6100=ORIENTED_EDGE('',*,*,#4711,.F.);
#6101=ORIENTED_EDGE('',*,*,#4707,.F.);
#6102=ORIENTED_EDGE('',*,*,#4712,.F.);
#6103=ORIENTED_EDGE('',*,*,#4713,.T.);
#6104=ORIENTED_EDGE('',*,*,#4714,.F.);
#6105=ORIENTED_EDGE('',*,*,#4710,.F.);
#6106=ORIENTED_EDGE('',*,*,#4715,.F.);
#6107=ORIENTED_EDGE('',*,*,#4716,.F.);
#6108=ORIENTED_EDGE('',*,*,#4717,.F.);
#6109=ORIENTED_EDGE('',*,*,#4713,.F.);
#6110=ORIENTED_EDGE('',*,*,#4718,.F.);
#6111=ORIENTED_EDGE('',*,*,#4719,.T.);
#6112=ORIENTED_EDGE('',*,*,#4720,.F.);
#6113=ORIENTED_EDGE('',*,*,#4721,.F.);
#6114=ORIENTED_EDGE('',*,*,#4722,.F.);
#6115=ORIENTED_EDGE('',*,*,#4723,.T.);
#6116=ORIENTED_EDGE('',*,*,#4724,.F.);
#6117=ORIENTED_EDGE('',*,*,#4719,.F.);
#6118=ORIENTED_EDGE('',*,*,#4725,.F.);
#6119=ORIENTED_EDGE('',*,*,#4726,.T.);
#6120=ORIENTED_EDGE('',*,*,#4727,.F.);
#6121=ORIENTED_EDGE('',*,*,#4723,.F.);
#6122=ORIENTED_EDGE('',*,*,#4728,.F.);
#6123=ORIENTED_EDGE('',*,*,#4729,.T.);
#6124=ORIENTED_EDGE('',*,*,#4730,.F.);
#6125=ORIENTED_EDGE('',*,*,#4726,.F.);
#6126=ORIENTED_EDGE('',*,*,#4731,.F.);
#6127=ORIENTED_EDGE('',*,*,#4732,.T.);
#6128=ORIENTED_EDGE('',*,*,#4733,.F.);
#6129=ORIENTED_EDGE('',*,*,#4729,.F.);
#6130=ORIENTED_EDGE('',*,*,#4734,.F.);
#6131=ORIENTED_EDGE('',*,*,#4735,.T.);
#6132=ORIENTED_EDGE('',*,*,#4736,.F.);
#6133=ORIENTED_EDGE('',*,*,#4732,.F.);
#6134=ORIENTED_EDGE('',*,*,#4737,.F.);
#6135=ORIENTED_EDGE('',*,*,#4738,.T.);
#6136=ORIENTED_EDGE('',*,*,#4739,.F.);
#6137=ORIENTED_EDGE('',*,*,#4735,.F.);
#6138=ORIENTED_EDGE('',*,*,#4740,.F.);
#6139=ORIENTED_EDGE('',*,*,#4741,.T.);
#6140=ORIENTED_EDGE('',*,*,#4742,.F.);
#6141=ORIENTED_EDGE('',*,*,#4738,.F.);
#6142=ORIENTED_EDGE('',*,*,#4743,.F.);
#6143=ORIENTED_EDGE('',*,*,#4744,.F.);
#6144=ORIENTED_EDGE('',*,*,#4745,.F.);
#6145=ORIENTED_EDGE('',*,*,#4741,.F.);
#6146=ORIENTED_EDGE('',*,*,#4746,.F.);
#6147=ORIENTED_EDGE('',*,*,#4747,.T.);
#6148=ORIENTED_EDGE('',*,*,#4748,.F.);
#6149=ORIENTED_EDGE('',*,*,#4747,.F.);
#6150=ORIENTED_EDGE('',*,*,#4660,.T.);
#6151=ORIENTED_EDGE('',*,*,#4749,.T.);
#6152=ORIENTED_EDGE('',*,*,#4750,.T.);
#6153=ORIENTED_EDGE('',*,*,#4751,.F.);
#6154=ORIENTED_EDGE('',*,*,#4637,.T.);
#6155=ORIENTED_EDGE('',*,*,#4752,.F.);
#6156=ORIENTED_EDGE('',*,*,#4753,.F.);
#6157=ORIENTED_EDGE('',*,*,#4754,.T.);
#6158=ORIENTED_EDGE('',*,*,#4688,.T.);
#6159=ORIENTED_EDGE('',*,*,#4755,.T.);
#6160=ORIENTED_EDGE('',*,*,#4753,.T.);
#6161=ORIENTED_EDGE('',*,*,#4756,.F.);
#6162=ORIENTED_EDGE('',*,*,#4665,.T.);
#6163=ORIENTED_EDGE('',*,*,#4757,.F.);
#6164=ORIENTED_EDGE('',*,*,#4758,.F.);
#6165=ORIENTED_EDGE('',*,*,#4759,.T.);
#6166=ORIENTED_EDGE('',*,*,#4716,.T.);
#6167=ORIENTED_EDGE('',*,*,#4760,.T.);
#6168=ORIENTED_EDGE('',*,*,#4758,.T.);
#6169=ORIENTED_EDGE('',*,*,#4761,.F.);
#6170=ORIENTED_EDGE('',*,*,#4693,.T.);
#6171=ORIENTED_EDGE('',*,*,#4762,.F.);
#6172=ORIENTED_EDGE('',*,*,#4763,.F.);
#6173=ORIENTED_EDGE('',*,*,#4764,.T.);
#6174=ORIENTED_EDGE('',*,*,#4744,.T.);
#6175=ORIENTED_EDGE('',*,*,#4765,.T.);
#6176=ORIENTED_EDGE('',*,*,#4763,.T.);
#6177=ORIENTED_EDGE('',*,*,#4766,.F.);
#6178=ORIENTED_EDGE('',*,*,#4721,.T.);
#6179=ORIENTED_EDGE('',*,*,#4767,.F.);
#6180=ORIENTED_EDGE('',*,*,#4750,.F.);
#6181=ORIENTED_EDGE('',*,*,#4768,.T.);
#6182=ORIENTED_EDGE('',*,*,#4636,.T.);
#6183=ORIENTED_EDGE('',*,*,#4640,.T.);
#6184=ORIENTED_EDGE('',*,*,#4643,.T.);
#6185=ORIENTED_EDGE('',*,*,#4646,.T.);
#6186=ORIENTED_EDGE('',*,*,#4649,.T.);
#6187=ORIENTED_EDGE('',*,*,#4652,.T.);
#6188=ORIENTED_EDGE('',*,*,#4655,.T.);
#6189=ORIENTED_EDGE('',*,*,#4658,.T.);
#6190=ORIENTED_EDGE('',*,*,#4661,.T.);
#6191=ORIENTED_EDGE('',*,*,#4751,.T.);
#6192=ORIENTED_EDGE('',*,*,#4767,.T.);
#6193=ORIENTED_EDGE('',*,*,#4720,.T.);
#6194=ORIENTED_EDGE('',*,*,#4724,.T.);
#6195=ORIENTED_EDGE('',*,*,#4727,.T.);
#6196=ORIENTED_EDGE('',*,*,#4730,.T.);
#6197=ORIENTED_EDGE('',*,*,#4733,.T.);
#6198=ORIENTED_EDGE('',*,*,#4736,.T.);
#6199=ORIENTED_EDGE('',*,*,#4739,.T.);
#6200=ORIENTED_EDGE('',*,*,#4742,.T.);
#6201=ORIENTED_EDGE('',*,*,#4745,.T.);
#6202=ORIENTED_EDGE('',*,*,#4766,.T.);
#6203=ORIENTED_EDGE('',*,*,#4762,.T.);
#6204=ORIENTED_EDGE('',*,*,#4692,.T.);
#6205=ORIENTED_EDGE('',*,*,#4696,.T.);
#6206=ORIENTED_EDGE('',*,*,#4699,.T.);
#6207=ORIENTED_EDGE('',*,*,#4702,.T.);
#6208=ORIENTED_EDGE('',*,*,#4705,.T.);
#6209=ORIENTED_EDGE('',*,*,#4708,.T.);
#6210=ORIENTED_EDGE('',*,*,#4711,.T.);
#6211=ORIENTED_EDGE('',*,*,#4714,.T.);
#6212=ORIENTED_EDGE('',*,*,#4717,.T.);
#6213=ORIENTED_EDGE('',*,*,#4761,.T.);
#6214=ORIENTED_EDGE('',*,*,#4757,.T.);
#6215=ORIENTED_EDGE('',*,*,#4664,.T.);
#6216=ORIENTED_EDGE('',*,*,#4668,.T.);
#6217=ORIENTED_EDGE('',*,*,#4671,.T.);
#6218=ORIENTED_EDGE('',*,*,#4674,.T.);
#6219=ORIENTED_EDGE('',*,*,#4677,.T.);
#6220=ORIENTED_EDGE('',*,*,#4680,.T.);
#6221=ORIENTED_EDGE('',*,*,#4683,.T.);
#6222=ORIENTED_EDGE('',*,*,#4686,.T.);
#6223=ORIENTED_EDGE('',*,*,#4689,.T.);
#6224=ORIENTED_EDGE('',*,*,#4756,.T.);
#6225=ORIENTED_EDGE('',*,*,#4752,.T.);
#6226=ORIENTED_EDGE('',*,*,#4748,.T.);
#6227=ORIENTED_EDGE('',*,*,#4634,.T.);
#6228=ORIENTED_EDGE('',*,*,#4754,.F.);
#6229=ORIENTED_EDGE('',*,*,#4755,.F.);
#6230=ORIENTED_EDGE('',*,*,#4687,.T.);
#6231=ORIENTED_EDGE('',*,*,#4684,.T.);
#6232=ORIENTED_EDGE('',*,*,#4681,.T.);
#6233=ORIENTED_EDGE('',*,*,#4678,.T.);
#6234=ORIENTED_EDGE('',*,*,#4675,.T.);
#6235=ORIENTED_EDGE('',*,*,#4672,.T.);
#6236=ORIENTED_EDGE('',*,*,#4669,.T.);
#6237=ORIENTED_EDGE('',*,*,#4666,.T.);
#6238=ORIENTED_EDGE('',*,*,#4662,.T.);
#6239=ORIENTED_EDGE('',*,*,#4759,.F.);
#6240=ORIENTED_EDGE('',*,*,#4760,.F.);
#6241=ORIENTED_EDGE('',*,*,#4715,.T.);
#6242=ORIENTED_EDGE('',*,*,#4712,.T.);
#6243=ORIENTED_EDGE('',*,*,#4709,.T.);
#6244=ORIENTED_EDGE('',*,*,#4706,.T.);
#6245=ORIENTED_EDGE('',*,*,#4703,.T.);
#6246=ORIENTED_EDGE('',*,*,#4700,.T.);
#6247=ORIENTED_EDGE('',*,*,#4697,.T.);
#6248=ORIENTED_EDGE('',*,*,#4694,.T.);
#6249=ORIENTED_EDGE('',*,*,#4690,.T.);
#6250=ORIENTED_EDGE('',*,*,#4764,.F.);
#6251=ORIENTED_EDGE('',*,*,#4765,.F.);
#6252=ORIENTED_EDGE('',*,*,#4743,.T.);
#6253=ORIENTED_EDGE('',*,*,#4740,.T.);
#6254=ORIENTED_EDGE('',*,*,#4737,.T.);
#6255=ORIENTED_EDGE('',*,*,#4734,.T.);
#6256=ORIENTED_EDGE('',*,*,#4731,.T.);
#6257=ORIENTED_EDGE('',*,*,#4728,.T.);
#6258=ORIENTED_EDGE('',*,*,#4725,.T.);
#6259=ORIENTED_EDGE('',*,*,#4722,.T.);
#6260=ORIENTED_EDGE('',*,*,#4718,.T.);
#6261=ORIENTED_EDGE('',*,*,#4768,.F.);
#6262=ORIENTED_EDGE('',*,*,#4749,.F.);
#6263=ORIENTED_EDGE('',*,*,#4659,.T.);
#6264=ORIENTED_EDGE('',*,*,#4656,.T.);
#6265=ORIENTED_EDGE('',*,*,#4653,.T.);
#6266=ORIENTED_EDGE('',*,*,#4650,.T.);
#6267=ORIENTED_EDGE('',*,*,#4647,.T.);
#6268=ORIENTED_EDGE('',*,*,#4644,.T.);
#6269=ORIENTED_EDGE('',*,*,#4641,.T.);
#6270=ORIENTED_EDGE('',*,*,#4638,.T.);
#6271=ORIENTED_EDGE('',*,*,#4746,.T.);
#7146=CYLINDRICAL_SURFACE('',#8308,0.21);
#7366=ADVANCED_FACE('',(#1098),#734,.F.);
#7367=ADVANCED_FACE('',(#1099),#735,.F.);
#7368=ADVANCED_FACE('',(#1100),#736,.F.);
#7369=ADVANCED_FACE('',(#1101),#737,.F.);
#7370=ADVANCED_FACE('',(#1102),#738,.F.);
#7371=ADVANCED_FACE('',(#1103),#739,.F.);
#7372=ADVANCED_FACE('',(#1104),#740,.F.);
#7373=ADVANCED_FACE('',(#1105),#741,.F.);
#7374=ADVANCED_FACE('',(#1106),#742,.F.);
#7375=ADVANCED_FACE('',(#1107),#743,.F.);
#7376=ADVANCED_FACE('',(#1108),#744,.F.);
#7377=ADVANCED_FACE('',(#1109),#745,.F.);
#7378=ADVANCED_FACE('',(#1110),#746,.F.);
#7379=ADVANCED_FACE('',(#1111),#747,.F.);
#7380=ADVANCED_FACE('',(#1112),#748,.F.);
#7381=ADVANCED_FACE('',(#1113),#749,.F.);
#7382=ADVANCED_FACE('',(#1114),#750,.F.);
#7383=ADVANCED_FACE('',(#1115),#751,.F.);
#7384=ADVANCED_FACE('',(#1116),#752,.F.);
#7385=ADVANCED_FACE('',(#1117),#753,.F.);
#7386=ADVANCED_FACE('',(#1118),#754,.F.);
#7387=ADVANCED_FACE('',(#1119),#755,.F.);
#7388=ADVANCED_FACE('',(#1120),#756,.F.);
#7389=ADVANCED_FACE('',(#1121),#757,.F.);
#7390=ADVANCED_FACE('',(#1122),#758,.F.);
#7391=ADVANCED_FACE('',(#1123),#759,.F.);
#7392=ADVANCED_FACE('',(#1124),#760,.F.);
#7393=ADVANCED_FACE('',(#1125),#761,.F.);
#7394=ADVANCED_FACE('',(#1126),#762,.F.);
#7395=ADVANCED_FACE('',(#1127),#763,.F.);
#7396=ADVANCED_FACE('',(#1128),#764,.F.);
#7397=ADVANCED_FACE('',(#1129),#765,.F.);
#7398=ADVANCED_FACE('',(#1130),#766,.F.);
#7399=ADVANCED_FACE('',(#1131),#767,.F.);
#7400=ADVANCED_FACE('',(#1132),#768,.F.);
#7401=ADVANCED_FACE('',(#1133),#769,.F.);
#7402=ADVANCED_FACE('',(#1134),#7146,.F.);
#7403=ADVANCED_FACE('',(#1135),#770,.T.);
#7404=ADVANCED_FACE('',(#1136),#771,.T.);
#7405=ADVANCED_FACE('',(#1137),#772,.T.);
#7406=ADVANCED_FACE('',(#1138),#773,.T.);
#7407=ADVANCED_FACE('',(#1139),#774,.T.);
#7408=ADVANCED_FACE('',(#1140),#775,.T.);
#7409=ADVANCED_FACE('',(#1141),#776,.T.);
#7410=ADVANCED_FACE('',(#1142),#777,.T.);
#7411=ADVANCED_FACE('',(#1143,#550),#778,.T.);
#7412=ADVANCED_FACE('',(#1144,#551),#779,.F.);
#7616=CLOSED_SHELL('',(#7366,#7367,#7368,#7369,#7370,#7371,#7372,#7373,
#7374,#7375,#7376,#7377,#7378,#7379,#7380,#7381,#7382,#7383,#7384,#7385,
#7386,#7387,#7388,#7389,#7390,#7391,#7392,#7393,#7394,#7395,#7396,#7397,
#7398,#7399,#7400,#7401,#7402,#7403,#7404,#7405,#7406,#7407,#7408,#7409,
#7410,#7411,#7412));
#8271=AXIS2_PLACEMENT_3D('',#11784,#9596,#9597);
#8272=AXIS2_PLACEMENT_3D('',#11785,#9598,#9599);
#8273=AXIS2_PLACEMENT_3D('',#11794,#9604,#9605);
#8274=AXIS2_PLACEMENT_3D('',#11800,#9609,#9610);
#8275=AXIS2_PLACEMENT_3D('',#11806,#9614,#9615);
#8276=AXIS2_PLACEMENT_3D('',#11812,#9619,#9620);
#8277=AXIS2_PLACEMENT_3D('',#11818,#9624,#9625);
#8278=AXIS2_PLACEMENT_3D('',#11824,#9629,#9630);
#8279=AXIS2_PLACEMENT_3D('',#11830,#9634,#9635);
#8280=AXIS2_PLACEMENT_3D('',#11836,#9639,#9640);
#8281=AXIS2_PLACEMENT_3D('',#11842,#9644,#9645);
#8282=AXIS2_PLACEMENT_3D('',#11851,#9650,#9651);
#8283=AXIS2_PLACEMENT_3D('',#11857,#9655,#9656);
#8284=AXIS2_PLACEMENT_3D('',#11863,#9660,#9661);
#8285=AXIS2_PLACEMENT_3D('',#11869,#9665,#9666);
#8286=AXIS2_PLACEMENT_3D('',#11875,#9670,#9671);
#8287=AXIS2_PLACEMENT_3D('',#11881,#9675,#9676);
#8288=AXIS2_PLACEMENT_3D('',#11887,#9680,#9681);
#8289=AXIS2_PLACEMENT_3D('',#11893,#9685,#9686);
#8290=AXIS2_PLACEMENT_3D('',#11899,#9690,#9691);
#8291=AXIS2_PLACEMENT_3D('',#11908,#9696,#9697);
#8292=AXIS2_PLACEMENT_3D('',#11914,#9701,#9702);
#8293=AXIS2_PLACEMENT_3D('',#11920,#9706,#9707);
#8294=AXIS2_PLACEMENT_3D('',#11926,#9711,#9712);
#8295=AXIS2_PLACEMENT_3D('',#11932,#9716,#9717);
#8296=AXIS2_PLACEMENT_3D('',#11938,#9721,#9722);
#8297=AXIS2_PLACEMENT_3D('',#11944,#9726,#9727);
#8298=AXIS2_PLACEMENT_3D('',#11950,#9731,#9732);
#8299=AXIS2_PLACEMENT_3D('',#11956,#9736,#9737);
#8300=AXIS2_PLACEMENT_3D('',#11965,#9742,#9743);
#8301=AXIS2_PLACEMENT_3D('',#11971,#9747,#9748);
#8302=AXIS2_PLACEMENT_3D('',#11977,#9752,#9753);
#8303=AXIS2_PLACEMENT_3D('',#11983,#9757,#9758);
#8304=AXIS2_PLACEMENT_3D('',#11989,#9762,#9763);
#8305=AXIS2_PLACEMENT_3D('',#11995,#9767,#9768);
#8306=AXIS2_PLACEMENT_3D('',#12001,#9772,#9773);
#8307=AXIS2_PLACEMENT_3D('',#12007,#9777,#9778);
#8308=AXIS2_PLACEMENT_3D('',#12013,#9782,#9783);
#8309=AXIS2_PLACEMENT_3D('',#12015,#9784,#9785);
#8310=AXIS2_PLACEMENT_3D('',#12018,#9787,#9788);
#8311=AXIS2_PLACEMENT_3D('',#12019,#9789,#9790);
#8312=AXIS2_PLACEMENT_3D('',#12025,#9794,#9795);
#8313=AXIS2_PLACEMENT_3D('',#12031,#9799,#9800);
#8314=AXIS2_PLACEMENT_3D('',#12034,#9803,#9804);
#8315=AXIS2_PLACEMENT_3D('',#12040,#9808,#9809);
#8316=AXIS2_PLACEMENT_3D('',#12043,#9812,#9813);
#8317=AXIS2_PLACEMENT_3D('',#12049,#9817,#9818);
#8318=AXIS2_PLACEMENT_3D('',#12052,#9821,#9822);
#8319=AXIS2_PLACEMENT_3D('',#12055,#9825,#9826);
#8320=AXIS2_PLACEMENT_3D('',#12056,#9827,#9828);
#9596=DIRECTION('axis',(0.,0.,1.));
#9597=DIRECTION('refdir',(1.,0.,0.));
#9598=DIRECTION('center_axis',(0.,0.,-1.));
#9599=DIRECTION('ref_axis',(0.,1.,0.));
#9600=DIRECTION('',(0.,1.,0.));
#9601=DIRECTION('',(1.,0.,0.));
#9602=DIRECTION('',(0.,-1.,0.));
#9603=DIRECTION('',(1.,0.,0.));
#9604=DIRECTION('center_axis',(0.,1.,-8.88178419700125E-16));
#9605=DIRECTION('ref_axis',(0.,8.88178419700125E-16,1.));
#9606=DIRECTION('',(0.,8.88178419700125E-16,1.));
#9607=DIRECTION('',(1.,0.,0.));
#9608=DIRECTION('',(0.,-8.88178419700125E-16,-1.));
#9609=DIRECTION('center_axis',(0.,-7.40148683083439E-16,-1.));
#9610=DIRECTION('ref_axis',(0.,1.,-7.40148683083439E-16));
#9611=DIRECTION('',(0.,1.,-7.40148683083439E-16));
#9612=DIRECTION('',(1.,0.,0.));
#9613=DIRECTION('',(0.,-1.,7.40148683083439E-16));
#9614=DIRECTION('center_axis',(0.,-0.707106781186547,-0.707106781186548));
#9615=DIRECTION('ref_axis',(0.,0.707106781186548,-0.707106781186547));
#9616=DIRECTION('',(0.,0.707106781186548,-0.707106781186547));
#9617=DIRECTION('',(1.,0.,0.));
#9618=DIRECTION('',(0.,-0.707106781186548,0.707106781186547));
#9619=DIRECTION('center_axis',(0.,-1.,2.77555756156289E-16));
#9620=DIRECTION('ref_axis',(0.,-2.77555756156289E-16,-1.));
#9621=DIRECTION('',(0.,-2.77555756156289E-16,-1.));
#9622=DIRECTION('',(1.,0.,0.));
#9623=DIRECTION('',(0.,2.77555756156289E-16,1.));
#9624=DIRECTION('center_axis',(0.,-0.707106781186547,0.707106781186548));
#9625=DIRECTION('ref_axis',(0.,-0.707106781186548,-0.707106781186547));
#9626=DIRECTION('',(0.,-0.707106781186548,-0.707106781186547));
#9627=DIRECTION('',(1.,0.,0.));
#9628=DIRECTION('',(0.,0.707106781186548,0.707106781186547));
#9629=DIRECTION('center_axis',(0.,7.40148683083438E-16,1.));
#9630=DIRECTION('ref_axis',(0.,-1.,7.40148683083438E-16));
#9631=DIRECTION('',(0.,-1.,7.40148683083438E-16));
#9632=DIRECTION('',(1.,0.,0.));
#9633=DIRECTION('',(0.,1.,-7.40148683083438E-16));
#9634=DIRECTION('center_axis',(0.,1.,-4.44089209850063E-16));
#9635=DIRECTION('ref_axis',(0.,4.44089209850063E-16,1.));
#9636=DIRECTION('',(0.,4.44089209850063E-16,1.));
#9637=DIRECTION('',(1.,0.,0.));
#9638=DIRECTION('',(0.,-4.44089209850063E-16,-1.));
#9639=DIRECTION('center_axis',(0.,2.41352831440251E-16,1.));
#9640=DIRECTION('ref_axis',(0.,-1.,2.41352831440251E-16));
#9641=DIRECTION('',(0.,-1.,2.41352831440251E-16));
#9642=DIRECTION('',(-1.,0.,0.));
#9643=DIRECTION('',(0.,1.,-2.41352831440251E-16));
#9644=DIRECTION('center_axis',(0.,-1.,2.41352831440251E-16));
#9645=DIRECTION('ref_axis',(0.,-2.41352831440251E-16,-1.));
#9646=DIRECTION('',(0.,-2.41352831440251E-16,-1.));
#9647=DIRECTION('',(1.,0.,0.));
#9648=DIRECTION('',(0.,2.41352831440251E-16,1.));
#9649=DIRECTION('',(1.,0.,0.));
#9650=DIRECTION('center_axis',(0.,0.,-1.));
#9651=DIRECTION('ref_axis',(0.,1.,0.));
#9652=DIRECTION('',(0.,1.,0.));
#9653=DIRECTION('',(1.,0.,0.));
#9654=DIRECTION('',(0.,-1.,0.));
#9655=DIRECTION('center_axis',(0.,-1.,0.));
#9656=DIRECTION('ref_axis',(0.,0.,-1.));
#9657=DIRECTION('',(0.,0.,-1.));
#9658=DIRECTION('',(1.,0.,0.));
#9659=DIRECTION('',(0.,0.,1.));
#9660=DIRECTION('center_axis',(0.,-0.707106781186547,0.707106781186548));
#9661=DIRECTION('ref_axis',(0.,-0.707106781186548,-0.707106781186547));
#9662=DIRECTION('',(0.,-0.707106781186548,-0.707106781186547));
#9663=DIRECTION('',(1.,0.,0.));
#9664=DIRECTION('',(0.,0.707106781186548,0.707106781186547));
#9665=DIRECTION('center_axis',(0.,0.,1.));
#9666=DIRECTION('ref_axis',(0.,-1.,0.));
#9667=DIRECTION('',(0.,-1.,0.));
#9668=DIRECTION('',(1.,0.,0.));
#9669=DIRECTION('',(0.,1.,0.));
#9670=DIRECTION('center_axis',(0.,0.707106781186548,0.707106781186547));
#9671=DIRECTION('ref_axis',(0.,-0.707106781186547,0.707106781186548));
#9672=DIRECTION('',(0.,-0.707106781186547,0.707106781186548));
#9673=DIRECTION('',(1.,0.,0.));
#9674=DIRECTION('',(0.,0.707106781186547,-0.707106781186548));
#9675=DIRECTION('center_axis',(0.,1.,0.));
#9676=DIRECTION('ref_axis',(0.,0.,1.));
#9677=DIRECTION('',(0.,0.,1.));
#9678=DIRECTION('',(1.,0.,0.));
#9679=DIRECTION('',(0.,0.,-1.));
#9680=DIRECTION('center_axis',(0.,0.,-1.));
#9681=DIRECTION('ref_axis',(0.,1.,0.));
#9682=DIRECTION('',(0.,1.,0.));
#9683=DIRECTION('',(1.,0.,0.));
#9684=DIRECTION('',(0.,-1.,0.));
#9685=DIRECTION('center_axis',(0.,1.,-2.41352831440251E-16));
#9686=DIRECTION('ref_axis',(0.,2.41352831440251E-16,1.));
#9687=DIRECTION('',(0.,2.41352831440251E-16,1.));
#9688=DIRECTION('',(-1.,0.,0.));
#9689=DIRECTION('',(0.,-2.41352831440251E-16,-1.));
#9690=DIRECTION('center_axis',(0.,0.,1.));
#9691=DIRECTION('ref_axis',(0.,-1.,0.));
#9692=DIRECTION('',(0.,-1.,0.));
#9693=DIRECTION('',(1.,0.,0.));
#9694=DIRECTION('',(0.,1.,0.));
#9695=DIRECTION('',(1.,0.,0.));
#9696=DIRECTION('center_axis',(0.,-1.,0.));
#9697=DIRECTION('ref_axis',(0.,0.,-1.));
#9698=DIRECTION('',(0.,0.,-1.));
#9699=DIRECTION('',(1.,0.,0.));
#9700=DIRECTION('',(0.,0.,1.));
#9701=DIRECTION('center_axis',(0.,0.,1.));
#9702=DIRECTION('ref_axis',(0.,-1.,0.));
#9703=DIRECTION('',(0.,-1.,0.));
#9704=DIRECTION('',(1.,0.,0.));
#9705=DIRECTION('',(0.,1.,0.));
#9706=DIRECTION('center_axis',(0.,0.707106781186548,0.707106781186548));
#9707=DIRECTION('ref_axis',(0.,-0.707106781186548,0.707106781186548));
#9708=DIRECTION('',(0.,-0.707106781186548,0.707106781186548));
#9709=DIRECTION('',(1.,0.,0.));
#9710=DIRECTION('',(0.,0.707106781186548,-0.707106781186548));
#9711=DIRECTION('center_axis',(0.,1.,0.));
#9712=DIRECTION('ref_axis',(0.,0.,1.));
#9713=DIRECTION('',(0.,0.,1.));
#9714=DIRECTION('',(1.,0.,0.));
#9715=DIRECTION('',(0.,0.,-1.));
#9716=DIRECTION('center_axis',(0.,0.707106781186548,-0.707106781186547));
#9717=DIRECTION('ref_axis',(0.,0.707106781186547,0.707106781186548));
#9718=DIRECTION('',(0.,0.707106781186547,0.707106781186548));
#9719=DIRECTION('',(1.,0.,0.));
#9720=DIRECTION('',(0.,-0.707106781186547,-0.707106781186548));
#9721=DIRECTION('center_axis',(0.,-7.40148683083438E-16,-1.));
#9722=DIRECTION('ref_axis',(0.,1.,-7.40148683083438E-16));
#9723=DIRECTION('',(0.,1.,-7.40148683083438E-16));
#9724=DIRECTION('',(1.,0.,0.));
#9725=DIRECTION('',(0.,-1.,7.40148683083438E-16));
#9726=DIRECTION('center_axis',(0.,-1.,0.));
#9727=DIRECTION('ref_axis',(0.,0.,-1.));
#9728=DIRECTION('',(0.,0.,-1.));
#9729=DIRECTION('',(1.,0.,0.));
#9730=DIRECTION('',(0.,0.,1.));
#9731=DIRECTION('center_axis',(0.,0.,-1.));
#9732=DIRECTION('ref_axis',(0.,1.,0.));
#9733=DIRECTION('',(0.,1.,0.));
#9734=DIRECTION('',(-1.,0.,0.));
#9735=DIRECTION('',(0.,-1.,0.));
#9736=DIRECTION('center_axis',(0.,1.,0.));
#9737=DIRECTION('ref_axis',(0.,0.,1.));
#9738=DIRECTION('',(0.,0.,1.));
#9739=DIRECTION('',(1.,0.,0.));
#9740=DIRECTION('',(0.,0.,-1.));
#9741=DIRECTION('',(1.,0.,0.));
#9742=DIRECTION('center_axis',(0.,0.,1.));
#9743=DIRECTION('ref_axis',(0.,-1.,0.));
#9744=DIRECTION('',(0.,-1.,0.));
#9745=DIRECTION('',(1.,0.,0.));
#9746=DIRECTION('',(0.,1.,0.));
#9747=DIRECTION('center_axis',(0.,1.,0.));
#9748=DIRECTION('ref_axis',(0.,0.,1.));
#9749=DIRECTION('',(0.,0.,1.));
#9750=DIRECTION('',(1.,0.,0.));
#9751=DIRECTION('',(0.,0.,-1.));
#9752=DIRECTION('center_axis',(0.,0.707106781186547,-0.707106781186548));
#9753=DIRECTION('ref_axis',(0.,0.707106781186548,0.707106781186547));
#9754=DIRECTION('',(0.,0.707106781186548,0.707106781186547));
#9755=DIRECTION('',(1.,0.,0.));
#9756=DIRECTION('',(0.,-0.707106781186548,-0.707106781186547));
#9757=DIRECTION('center_axis',(0.,0.,-1.));
#9758=DIRECTION('ref_axis',(0.,1.,0.));
#9759=DIRECTION('',(0.,1.,0.));
#9760=DIRECTION('',(1.,0.,0.));
#9761=DIRECTION('',(0.,-1.,0.));
#9762=DIRECTION('center_axis',(0.,-0.707106781186547,-0.707106781186548));
#9763=DIRECTION('ref_axis',(0.,0.707106781186548,-0.707106781186547));
#9764=DIRECTION('',(0.,0.707106781186548,-0.707106781186547));
#9765=DIRECTION('',(1.,0.,0.));
#9766=DIRECTION('',(0.,-0.707106781186548,0.707106781186547));
#9767=DIRECTION('center_axis',(0.,-1.,0.));
#9768=DIRECTION('ref_axis',(0.,0.,-1.));
#9769=DIRECTION('',(0.,0.,-1.));
#9770=DIRECTION('',(1.,0.,0.));
#9771=DIRECTION('',(0.,0.,1.));
#9772=DIRECTION('center_axis',(0.,0.,1.));
#9773=DIRECTION('ref_axis',(0.,-1.,0.));
#9774=DIRECTION('',(0.,-1.,0.));
#9775=DIRECTION('',(1.,0.,0.));
#9776=DIRECTION('',(0.,1.,0.));
#9777=DIRECTION('center_axis',(0.,-1.,0.));
#9778=DIRECTION('ref_axis',(0.,0.,-1.));
#9779=DIRECTION('',(0.,0.,-1.));
#9780=DIRECTION('',(-1.,0.,0.));
#9781=DIRECTION('',(0.,0.,1.));
#9782=DIRECTION('center_axis',(1.,0.,0.));
#9783=DIRECTION('ref_axis',(0.,0.,-1.));
#9784=DIRECTION('center_axis',(1.,0.,0.));
#9785=DIRECTION('ref_axis',(0.,0.,-1.));
#9786=DIRECTION('',(1.,0.,0.));
#9787=DIRECTION('center_axis',(-1.,0.,0.));
#9788=DIRECTION('ref_axis',(0.,0.,-1.));
#9789=DIRECTION('center_axis',(0.,1.,0.));
#9790=DIRECTION('ref_axis',(0.,0.,1.));
#9791=DIRECTION('',(0.,0.,1.));
#9792=DIRECTION('',(1.,0.,0.));
#9793=DIRECTION('',(0.,0.,1.));
#9794=DIRECTION('center_axis',(0.,1.,0.));
#9795=DIRECTION('ref_axis',(0.,0.,1.));
#9796=DIRECTION('',(0.,0.,1.));
#9797=DIRECTION('',(1.,0.,0.));
#9798=DIRECTION('',(0.,0.,1.));
#9799=DIRECTION('center_axis',(0.,0.,-1.));
#9800=DIRECTION('ref_axis',(0.,1.,0.));
#9801=DIRECTION('',(0.,1.,0.));
#9802=DIRECTION('',(0.,1.,0.));
#9803=DIRECTION('center_axis',(0.,0.,-1.));
#9804=DIRECTION('ref_axis',(0.,1.,0.));
#9805=DIRECTION('',(0.,1.,0.));
#9806=DIRECTION('',(1.,0.,0.));
#9807=DIRECTION('',(0.,1.,0.));
#9808=DIRECTION('center_axis',(0.,-1.,0.));
#9809=DIRECTION('ref_axis',(0.,0.,-1.));
#9810=DIRECTION('',(0.,0.,-1.));
#9811=DIRECTION('',(0.,0.,-1.));
#9812=DIRECTION('center_axis',(0.,-1.,0.));
#9813=DIRECTION('ref_axis',(0.,0.,-1.));
#9814=DIRECTION('',(0.,0.,-1.));
#9815=DIRECTION('',(1.,0.,0.));
#9816=DIRECTION('',(0.,0.,-1.));
#9817=DIRECTION('center_axis',(0.,0.,1.));
#9818=DIRECTION('ref_axis',(0.,-1.,0.));
#9819=DIRECTION('',(0.,-1.,0.));
#9820=DIRECTION('',(0.,-1.,0.));
#9821=DIRECTION('center_axis',(0.,0.,1.));
#9822=DIRECTION('ref_axis',(0.,-1.,0.));
#9823=DIRECTION('',(0.,-1.,0.));
#9824=DIRECTION('',(0.,-1.,0.));
#9825=DIRECTION('center_axis',(1.,0.,0.));
#9826=DIRECTION('ref_axis',(0.,0.,-1.));
#9827=DIRECTION('center_axis',(1.,0.,0.));
#9828=DIRECTION('ref_axis',(0.,0.,-1.));
#11784=CARTESIAN_POINT('',(0.,0.,0.));
#11785=CARTESIAN_POINT('Origin',(-0.1,0.82,-0.3));
#11786=CARTESIAN_POINT('',(0.,0.82,-0.3));
#11787=CARTESIAN_POINT('',(0.,1.,-0.3));
#11788=CARTESIAN_POINT('',(0.,0.41,-0.3));
#11789=CARTESIAN_POINT('',(40.,0.82,-0.3));
#11790=CARTESIAN_POINT('',(-0.1,0.82,-0.3));
#11791=CARTESIAN_POINT('',(40.,1.,-0.3));
#11792=CARTESIAN_POINT('',(40.,0.41,-0.3));
#11793=CARTESIAN_POINT('',(-0.05,1.,-0.3));
#11794=CARTESIAN_POINT('Origin',(-0.1,0.82,-0.55));
#11795=CARTESIAN_POINT('',(0.,0.82,-0.55));
#11796=CARTESIAN_POINT('',(0.,0.82,-0.275));
#11797=CARTESIAN_POINT('',(40.,0.82,-0.55));
#11798=CARTESIAN_POINT('',(-0.1,0.82,-0.55));
#11799=CARTESIAN_POINT('',(40.,0.82,-0.275));
#11800=CARTESIAN_POINT('Origin',(-0.1,0.67,-0.55));
#11801=CARTESIAN_POINT('',(0.,0.67,-0.55));
#11802=CARTESIAN_POINT('',(0.,0.335,-0.55));
#11803=CARTESIAN_POINT('',(40.,0.67,-0.55));
#11804=CARTESIAN_POINT('',(-0.1,0.67,-0.55));
#11805=CARTESIAN_POINT('',(40.,0.335,-0.55));
#11806=CARTESIAN_POINT('Origin',(-0.1,0.42,-0.3));
#11807=CARTESIAN_POINT('',(0.,0.42,-0.3));
#11808=CARTESIAN_POINT('',(0.,0.24,-0.12));
#11809=CARTESIAN_POINT('',(40.,0.42,-0.3));
#11810=CARTESIAN_POINT('',(-0.1,0.42,-0.3));
#11811=CARTESIAN_POINT('',(40.,0.24,-0.12));
#11812=CARTESIAN_POINT('Origin',(-0.1,0.42,0.3));
#11813=CARTESIAN_POINT('',(0.,0.42,0.3));
#11814=CARTESIAN_POINT('',(0.,0.42,0.15));
#11815=CARTESIAN_POINT('',(40.,0.42,0.3));
#11816=CARTESIAN_POINT('',(-0.1,0.42,0.3));
#11817=CARTESIAN_POINT('',(40.,0.42,0.15));
#11818=CARTESIAN_POINT('Origin',(-0.1,0.67,0.55));
#11819=CARTESIAN_POINT('',(0.,0.67,0.55));
#11820=CARTESIAN_POINT('',(6.93889390390723E-18,0.365,0.245));
#11821=CARTESIAN_POINT('',(40.,0.67,0.55));
#11822=CARTESIAN_POINT('',(-0.1,0.67,0.55));
#11823=CARTESIAN_POINT('',(40.,0.365,0.245));
#11824=CARTESIAN_POINT('Origin',(-0.1,0.82,0.55));
#11825=CARTESIAN_POINT('',(0.,0.82,0.55));
#11826=CARTESIAN_POINT('',(0.,0.41,0.55));
#11827=CARTESIAN_POINT('',(40.,0.82,0.55));
#11828=CARTESIAN_POINT('',(-0.1,0.82,0.55));
#11829=CARTESIAN_POINT('',(40.,0.41,0.55));
#11830=CARTESIAN_POINT('Origin',(-0.1,0.82,0.3));
#11831=CARTESIAN_POINT('',(0.,0.82,0.3));
#11832=CARTESIAN_POINT('',(0.,0.82,0.15));
#11833=CARTESIAN_POINT('',(40.,0.82,0.3));
#11834=CARTESIAN_POINT('',(-0.1,0.82,0.3));
#11835=CARTESIAN_POINT('',(40.,0.82,0.15));
#11836=CARTESIAN_POINT('Origin',(-0.1,1.05,0.3));
#11837=CARTESIAN_POINT('',(0.,1.,0.3));
#11838=CARTESIAN_POINT('',(0.,0.525,0.3));
#11839=CARTESIAN_POINT('',(40.,1.,0.3));
#11840=CARTESIAN_POINT('',(-0.05,1.,0.3));
#11841=CARTESIAN_POINT('',(40.,0.525,0.3));
#11842=CARTESIAN_POINT('Origin',(-0.1,-0.3,-0.82));
#11843=CARTESIAN_POINT('',(0.,-0.3,-0.82));
#11844=CARTESIAN_POINT('',(0.,-0.3,-1.));
#11845=CARTESIAN_POINT('',(0.,-0.3,-0.41));
#11846=CARTESIAN_POINT('',(40.,-0.3,-0.82));
#11847=CARTESIAN_POINT('',(-0.1,-0.3,-0.82));
#11848=CARTESIAN_POINT('',(40.,-0.3,-1.));
#11849=CARTESIAN_POINT('',(40.,-0.3,-0.41));
#11850=CARTESIAN_POINT('',(-0.05,-0.3,-1.));
#11851=CARTESIAN_POINT('Origin',(-0.1,-0.55,-0.82));
#11852=CARTESIAN_POINT('',(0.,-0.55,-0.82));
#11853=CARTESIAN_POINT('',(0.,-0.275,-0.82));
#11854=CARTESIAN_POINT('',(40.,-0.55,-0.82));
#11855=CARTESIAN_POINT('',(-0.1,-0.55,-0.82));
#11856=CARTESIAN_POINT('',(40.,-0.275,-0.82));
#11857=CARTESIAN_POINT('Origin',(-0.1,-0.55,-0.67));
#11858=CARTESIAN_POINT('',(0.,-0.55,-0.67));
#11859=CARTESIAN_POINT('',(0.,-0.55,-0.335));
#11860=CARTESIAN_POINT('',(40.,-0.55,-0.67));
#11861=CARTESIAN_POINT('',(-0.1,-0.55,-0.67));
#11862=CARTESIAN_POINT('',(40.,-0.55,-0.335));
#11863=CARTESIAN_POINT('Origin',(-0.1,-0.3,-0.42));
#11864=CARTESIAN_POINT('',(0.,-0.3,-0.42));
#11865=CARTESIAN_POINT('',(0.,-0.12,-0.24));
#11866=CARTESIAN_POINT('',(40.,-0.3,-0.42));
#11867=CARTESIAN_POINT('',(-0.1,-0.3,-0.42));
#11868=CARTESIAN_POINT('',(40.,-0.12,-0.24));
#11869=CARTESIAN_POINT('Origin',(-0.1,0.3,-0.42));
#11870=CARTESIAN_POINT('',(0.,0.3,-0.42));
#11871=CARTESIAN_POINT('',(0.,0.15,-0.42));
#11872=CARTESIAN_POINT('',(40.,0.3,-0.42));
#11873=CARTESIAN_POINT('',(-0.1,0.3,-0.42));
#11874=CARTESIAN_POINT('',(40.,0.15,-0.42));
#11875=CARTESIAN_POINT('Origin',(-0.1,0.55,-0.67));
#11876=CARTESIAN_POINT('',(0.,0.55,-0.67));
#11877=CARTESIAN_POINT('',(0.,0.245,-0.365));
#11878=CARTESIAN_POINT('',(40.,0.55,-0.67));
#11879=CARTESIAN_POINT('',(-0.1,0.55,-0.67));
#11880=CARTESIAN_POINT('',(40.,0.245,-0.365));
#11881=CARTESIAN_POINT('Origin',(-0.1,0.55,-0.82));
#11882=CARTESIAN_POINT('',(0.,0.55,-0.82));
#11883=CARTESIAN_POINT('',(0.,0.55,-0.41));
#11884=CARTESIAN_POINT('',(40.,0.55,-0.82));
#11885=CARTESIAN_POINT('',(-0.1,0.55,-0.82));
#11886=CARTESIAN_POINT('',(40.,0.55,-0.41));
#11887=CARTESIAN_POINT('Origin',(-0.1,0.3,-0.82));
#11888=CARTESIAN_POINT('',(0.,0.3,-0.82));
#11889=CARTESIAN_POINT('',(0.,0.15,-0.82));
#11890=CARTESIAN_POINT('',(40.,0.3,-0.82));
#11891=CARTESIAN_POINT('',(-0.1,0.3,-0.82));
#11892=CARTESIAN_POINT('',(40.,0.15,-0.82));
#11893=CARTESIAN_POINT('Origin',(-0.1,0.3,-1.05));
#11894=CARTESIAN_POINT('',(0.,0.3,-1.));
#11895=CARTESIAN_POINT('',(0.,0.3,-0.525));
#11896=CARTESIAN_POINT('',(40.,0.3,-1.));
#11897=CARTESIAN_POINT('',(-0.05,0.3,-1.));
#11898=CARTESIAN_POINT('',(40.,0.3,-0.525));
#11899=CARTESIAN_POINT('Origin',(-0.1,-0.82,0.3));
#11900=CARTESIAN_POINT('',(0.,-0.82,0.3));
#11901=CARTESIAN_POINT('',(0.,-1.,0.3));
#11902=CARTESIAN_POINT('',(0.,-0.41,0.3));
#11903=CARTESIAN_POINT('',(40.,-0.82,0.3));
#11904=CARTESIAN_POINT('',(-0.1,-0.82,0.3));
#11905=CARTESIAN_POINT('',(40.,-1.,0.3));
#11906=CARTESIAN_POINT('',(40.,-0.41,0.3));
#11907=CARTESIAN_POINT('',(-0.05,-1.,0.3));
#11908=CARTESIAN_POINT('Origin',(-0.1,-0.82,0.55));
#11909=CARTESIAN_POINT('',(0.,-0.82,0.55));
#11910=CARTESIAN_POINT('',(0.,-0.82,0.275));
#11911=CARTESIAN_POINT('',(40.,-0.82,0.55));
#11912=CARTESIAN_POINT('',(-0.1,-0.82,0.55));
#11913=CARTESIAN_POINT('',(40.,-0.82,0.275));
#11914=CARTESIAN_POINT('Origin',(-0.1,-0.67,0.55));
#11915=CARTESIAN_POINT('',(0.,-0.67,0.55));
#11916=CARTESIAN_POINT('',(0.,-0.335,0.55));
#11917=CARTESIAN_POINT('',(40.,-0.67,0.55));
#11918=CARTESIAN_POINT('',(-0.1,-0.67,0.55));
#11919=CARTESIAN_POINT('',(40.,-0.335,0.55));
#11920=CARTESIAN_POINT('Origin',(-0.1,-0.42,0.3));
#11921=CARTESIAN_POINT('',(0.,-0.42,0.3));
#11922=CARTESIAN_POINT('',(-6.93889390390723E-18,-0.24,0.12));
#11923=CARTESIAN_POINT('',(40.,-0.42,0.3));
#11924=CARTESIAN_POINT('',(-0.1,-0.42,0.3));
#11925=CARTESIAN_POINT('',(40.,-0.24,0.12));
#11926=CARTESIAN_POINT('Origin',(-0.1,-0.42,-0.3));
#11927=CARTESIAN_POINT('',(0.,-0.42,-0.3));
#11928=CARTESIAN_POINT('',(0.,-0.42,-0.15));
#11929=CARTESIAN_POINT('',(40.,-0.42,-0.3));
#11930=CARTESIAN_POINT('',(-0.1,-0.42,-0.3));
#11931=CARTESIAN_POINT('',(40.,-0.42,-0.15));
#11932=CARTESIAN_POINT('Origin',(-0.1,-0.67,-0.55));
#11933=CARTESIAN_POINT('',(0.,-0.67,-0.55));
#11934=CARTESIAN_POINT('',(0.,-0.365,-0.245));
#11935=CARTESIAN_POINT('',(40.,-0.67,-0.55));
#11936=CARTESIAN_POINT('',(-0.1,-0.67,-0.55));
#11937=CARTESIAN_POINT('',(40.,-0.365,-0.245));
#11938=CARTESIAN_POINT('Origin',(-0.1,-0.82,-0.55));
#11939=CARTESIAN_POINT('',(0.,-0.82,-0.55));
#11940=CARTESIAN_POINT('',(0.,-0.41,-0.55));
#11941=CARTESIAN_POINT('',(40.,-0.82,-0.55));
#11942=CARTESIAN_POINT('',(-0.1,-0.82,-0.55));
#11943=CARTESIAN_POINT('',(40.,-0.41,-0.55));
#11944=CARTESIAN_POINT('Origin',(-0.1,-0.82,-0.3));
#11945=CARTESIAN_POINT('',(0.,-0.82,-0.3));
#11946=CARTESIAN_POINT('',(0.,-0.82,-0.15));
#11947=CARTESIAN_POINT('',(40.,-0.82,-0.3));
#11948=CARTESIAN_POINT('',(-0.1,-0.82,-0.3));
#11949=CARTESIAN_POINT('',(40.,-0.82,-0.15));
#11950=CARTESIAN_POINT('Origin',(-0.1,-1.05,-0.3));
#11951=CARTESIAN_POINT('',(0.,-1.,-0.3));
#11952=CARTESIAN_POINT('',(0.,-0.525,-0.3));
#11953=CARTESIAN_POINT('',(40.,-1.,-0.3));
#11954=CARTESIAN_POINT('',(-0.05,-1.,-0.3));
#11955=CARTESIAN_POINT('',(40.,-0.525,-0.3));
#11956=CARTESIAN_POINT('Origin',(-0.1,0.3,0.82));
#11957=CARTESIAN_POINT('',(0.,0.3,0.82));
#11958=CARTESIAN_POINT('',(0.,0.3,1.));
#11959=CARTESIAN_POINT('',(0.,0.3,0.41));
#11960=CARTESIAN_POINT('',(40.,0.3,0.82));
#11961=CARTESIAN_POINT('',(-0.1,0.3,0.82));
#11962=CARTESIAN_POINT('',(40.,0.3,1.));
#11963=CARTESIAN_POINT('',(40.,0.3,0.41));
#11964=CARTESIAN_POINT('',(-0.05,0.3,1.));
#11965=CARTESIAN_POINT('Origin',(-0.1,0.55,0.82));
#11966=CARTESIAN_POINT('',(0.,0.55,0.82));
#11967=CARTESIAN_POINT('',(0.,0.275,0.82));
#11968=CARTESIAN_POINT('',(40.,0.55,0.82));
#11969=CARTESIAN_POINT('',(-0.1,0.55,0.82));
#11970=CARTESIAN_POINT('',(40.,0.275,0.82));
#11971=CARTESIAN_POINT('Origin',(-0.1,0.55,0.67));
#11972=CARTESIAN_POINT('',(0.,0.55,0.67));
#11973=CARTESIAN_POINT('',(0.,0.55,0.335));
#11974=CARTESIAN_POINT('',(40.,0.55,0.67));
#11975=CARTESIAN_POINT('',(-0.1,0.55,0.67));
#11976=CARTESIAN_POINT('',(40.,0.55,0.335));
#11977=CARTESIAN_POINT('Origin',(-0.1,0.3,0.42));
#11978=CARTESIAN_POINT('',(0.,0.3,0.42));
#11979=CARTESIAN_POINT('',(6.93889390390723E-18,0.12,0.24));
#11980=CARTESIAN_POINT('',(40.,0.3,0.42));
#11981=CARTESIAN_POINT('',(-0.1,0.3,0.42));
#11982=CARTESIAN_POINT('',(40.,0.12,0.24));
#11983=CARTESIAN_POINT('Origin',(-0.1,-0.3,0.42));
#11984=CARTESIAN_POINT('',(0.,-0.3,0.42));
#11985=CARTESIAN_POINT('',(0.,-0.15,0.42));
#11986=CARTESIAN_POINT('',(40.,-0.3,0.42));
#11987=CARTESIAN_POINT('',(-0.1,-0.3,0.42));
#11988=CARTESIAN_POINT('',(40.,-0.15,0.42));
#11989=CARTESIAN_POINT('Origin',(-0.1,-0.55,0.67));
#11990=CARTESIAN_POINT('',(0.,-0.55,0.67));
#11991=CARTESIAN_POINT('',(6.93889390390723E-18,-0.245,0.365));
#11992=CARTESIAN_POINT('',(40.,-0.55,0.67));
#11993=CARTESIAN_POINT('',(-0.1,-0.55,0.67));
#11994=CARTESIAN_POINT('',(40.,-0.245,0.365));
#11995=CARTESIAN_POINT('Origin',(-0.1,-0.55,0.82));
#11996=CARTESIAN_POINT('',(0.,-0.55,0.82));
#11997=CARTESIAN_POINT('',(0.,-0.55,0.41));
#11998=CARTESIAN_POINT('',(40.,-0.55,0.82));
#11999=CARTESIAN_POINT('',(-0.1,-0.55,0.82));
#12000=CARTESIAN_POINT('',(40.,-0.55,0.41));
#12001=CARTESIAN_POINT('Origin',(-0.1,-0.3,0.82));
#12002=CARTESIAN_POINT('',(0.,-0.3,0.82));
#12003=CARTESIAN_POINT('',(0.,-0.15,0.82));
#12004=CARTESIAN_POINT('',(40.,-0.3,0.82));
#12005=CARTESIAN_POINT('',(-0.1,-0.3,0.82));
#12006=CARTESIAN_POINT('',(40.,-0.15,0.82));
#12007=CARTESIAN_POINT('Origin',(-0.1,-0.3,1.05));
#12008=CARTESIAN_POINT('',(0.,-0.3,1.));
#12009=CARTESIAN_POINT('',(0.,-0.3,0.525));
#12010=CARTESIAN_POINT('',(40.,-0.3,1.));
#12011=CARTESIAN_POINT('',(-0.05,-0.3,1.));
#12012=CARTESIAN_POINT('',(40.,-0.3,0.525));
#12013=CARTESIAN_POINT('Origin',(-0.1,0.,0.));
#12014=CARTESIAN_POINT('',(0.,-2.57175827820944E-17,0.21));
#12015=CARTESIAN_POINT('Origin',(0.,0.,0.));
#12016=CARTESIAN_POINT('',(40.,2.57175827820944E-17,0.21));
#12017=CARTESIAN_POINT('',(-0.1,-2.57175827820944E-17,0.21));
#12018=CARTESIAN_POINT('Origin',(40.,0.,0.));
#12019=CARTESIAN_POINT('Origin',(0.,1.,-1.));
#12020=CARTESIAN_POINT('',(0.,1.,1.));
#12021=CARTESIAN_POINT('',(0.,1.,-1.));
#12022=CARTESIAN_POINT('',(40.,1.,1.));
#12023=CARTESIAN_POINT('',(0.,1.,1.));
#12024=CARTESIAN_POINT('',(40.,1.,-1.));
#12025=CARTESIAN_POINT('Origin',(0.,1.,-1.));
#12026=CARTESIAN_POINT('',(40.,1.,-1.));
#12027=CARTESIAN_POINT('',(40.,1.,-1.));
#12028=CARTESIAN_POINT('',(0.,1.,-1.));
#12029=CARTESIAN_POINT('',(0.,1.,-1.));
#12030=CARTESIAN_POINT('',(0.,1.,-1.));
#12031=CARTESIAN_POINT('Origin',(0.,-1.,-1.));
#12032=CARTESIAN_POINT('',(0.,-1.,-1.));
#12033=CARTESIAN_POINT('',(40.,-1.,-1.));
#12034=CARTESIAN_POINT('Origin',(0.,-1.,-1.));
#12035=CARTESIAN_POINT('',(40.,-1.,-1.));
#12036=CARTESIAN_POINT('',(40.,-1.,-1.));
#12037=CARTESIAN_POINT('',(0.,-1.,-1.));
#12038=CARTESIAN_POINT('',(0.,-1.,-1.));
#12039=CARTESIAN_POINT('',(0.,-1.,-1.));
#12040=CARTESIAN_POINT('Origin',(0.,-1.,1.));
#12041=CARTESIAN_POINT('',(0.,-1.,1.));
#12042=CARTESIAN_POINT('',(40.,-1.,1.));
#12043=CARTESIAN_POINT('Origin',(0.,-1.,1.));
#12044=CARTESIAN_POINT('',(40.,-1.,1.));
#12045=CARTESIAN_POINT('',(40.,-1.,1.));
#12046=CARTESIAN_POINT('',(0.,-1.,1.));
#12047=CARTESIAN_POINT('',(0.,-1.,1.));
#12048=CARTESIAN_POINT('',(0.,-1.,1.));
#12049=CARTESIAN_POINT('Origin',(0.,1.,1.));
#12050=CARTESIAN_POINT('',(0.,1.,1.));
#12051=CARTESIAN_POINT('',(40.,1.,1.));
#12052=CARTESIAN_POINT('Origin',(0.,1.,1.));
#12053=CARTESIAN_POINT('',(40.,1.,1.));
#12054=CARTESIAN_POINT('',(0.,1.,1.));
#12055=CARTESIAN_POINT('Origin',(40.,0.,0.));
#12056=CARTESIAN_POINT('Origin',(0.,0.,0.));
#13042=UNCERTAINTY_MEASURE_WITH_UNIT(LENGTH_MEASURE(0.001),#13095,
'DISTANCE_ACCURACY_VALUE',
'Maximum model space distance between geometric entities at asserted c
onnectivities');
#13057=UNCERTAINTY_MEASURE_WITH_UNIT(LENGTH_MEASURE(0.001),#13095,
'DISTANCE_ACCURACY_VALUE',
'Maximum model space distance between geometric entities at asserted c
onnectivities');
#13079=(
GEOMETRIC_REPRESENTATION_CONTEXT(3)
GLOBAL_UNCERTAINTY_ASSIGNED_CONTEXT((#13042))
GLOBAL_UNIT_ASSIGNED_CONTEXT((#13095,#13097,#13098))
REPRESENTATION_CONTEXT('','3D')
);
#13094=(
GEOMETRIC_REPRESENTATION_CONTEXT(3)
GLOBAL_UNCERTAINTY_ASSIGNED_CONTEXT((#13057))
GLOBAL_UNIT_ASSIGNED_CONTEXT((#13095,#13097,#13098))
REPRESENTATION_CONTEXT('','3D')
);
#13095=(
LENGTH_UNIT()
NAMED_UNIT(*)
SI_UNIT(.CENTI.,.METRE.)
);
#13097=(
NAMED_UNIT(*)
PLANE_ANGLE_UNIT()
SI_UNIT($,.RADIAN.)
);
#13098=(
NAMED_UNIT(*)
SI_UNIT($,.STERADIAN.)
SOLID_ANGLE_UNIT()
);
#13120=SHAPE_DEFINITION_REPRESENTATION(#13156,#13270);
#13156=PRODUCT_DEFINITION_SHAPE('',$,#13307);
#13270=SHAPE_REPRESENTATION('',(#8271),#13079);
#13285=PRODUCT_DEFINITION_CONTEXT('part definition',#13395,'design');
#13307=PRODUCT_DEFINITION('Slotted Extrusion - 20 x 20 x 400 mm',
'Slotted Extrusion - 20 x 20 x 400 mm',#13343,#13285);
#13343=PRODUCT_DEFINITION_FORMATION('',$,#13418);
#13395=APPLICATION_CONTEXT(
'Core Data for Automotive Mechanical Design Process');
#13396=PRODUCT_CONTEXT('part definition',#13395,'mechanical');
#13418=PRODUCT('Slotted Extrusion - 20 x 20 x 400 mm',
'Slotted Extrusion - 20 x 20 x 400 mm',
'Slotted Extrusion - 20 x 20 x 400 mm',(#13396));
#13475=COLOUR_RGB('Light Blue',0.38,0.62,0.78);
#13476=FILL_AREA_STYLE_COLOUR('',#13475);
#13477=FILL_AREA_STYLE('',(#13476));
#13478=SURFACE_STYLE_FILL_AREA(#13477);
#13479=SURFACE_SIDE_STYLE('',(#13478));
#13480=SURFACE_STYLE_USAGE(.BOTH.,#13479);
#13481=PRESENTATION_STYLE_ASSIGNMENT((#13480));
ENDSEC;
END-ISO-10303-21;
